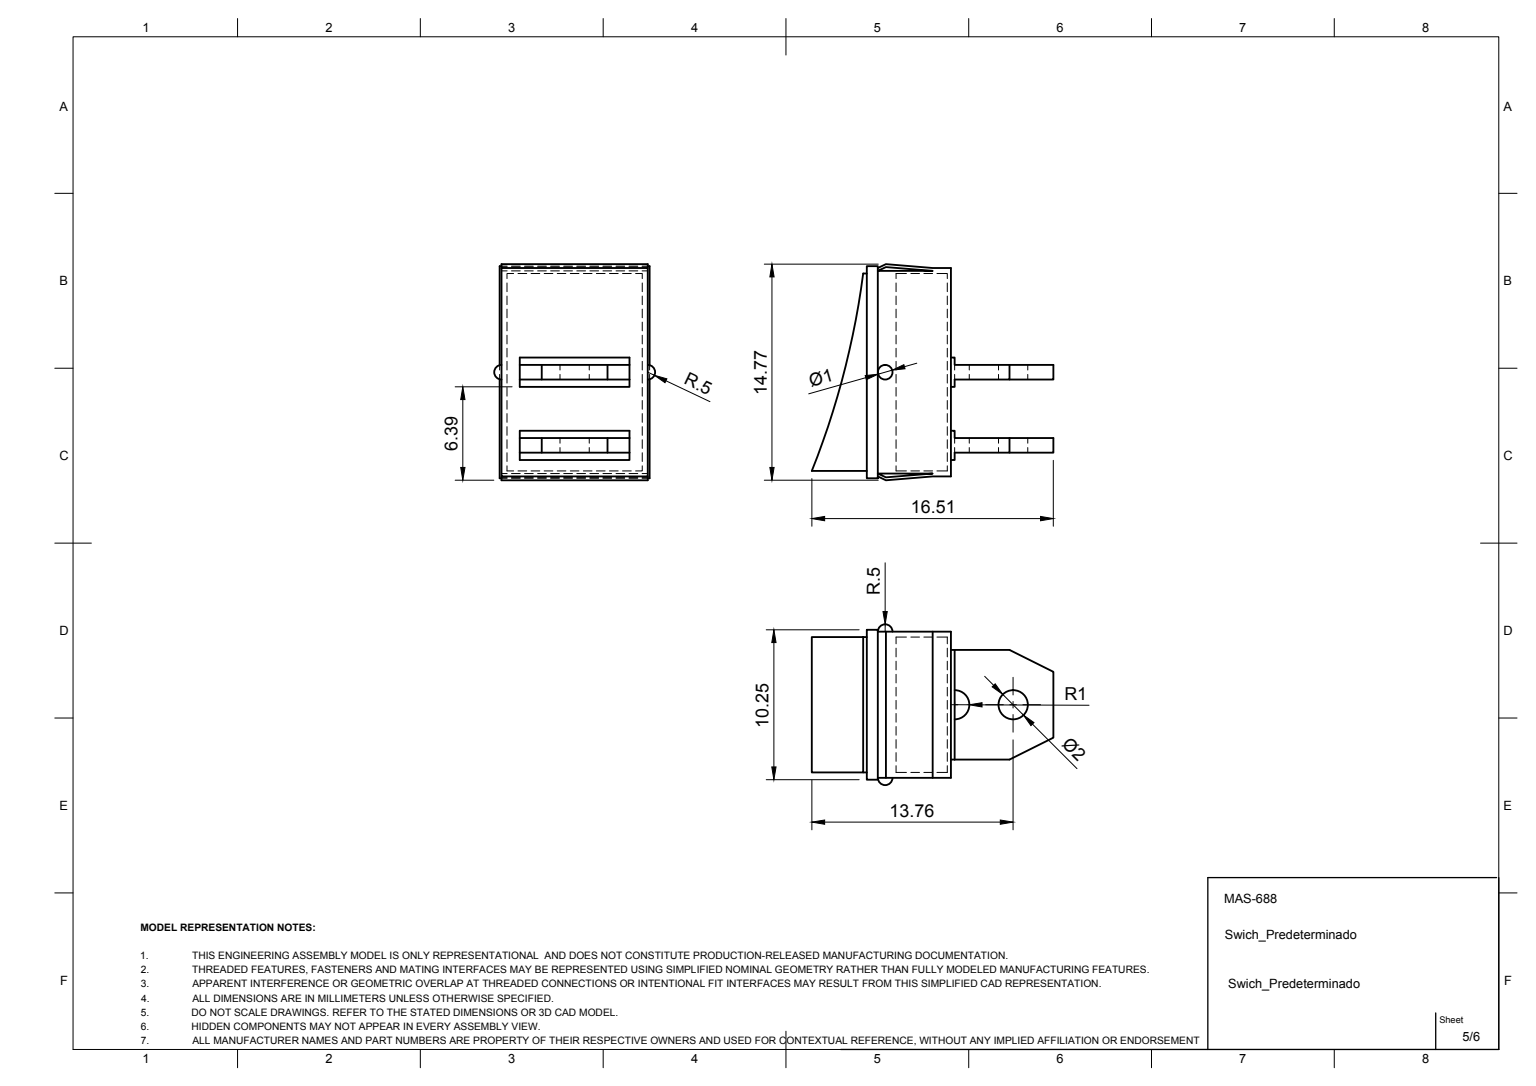
ISO-10303-21;
HEADER;
/* Generated by software containing ST-Developer
 * from STEP Tools, Inc. (www.steptools.com) 
 */

FILE_DESCRIPTION(
/* description */ ('STEP AP214'),
/* implementation_level */ '2;1');

FILE_NAME(
/* name */ 'Swich_Predeterminado.step',
/* time_stamp */ '2026-11-14T03:58:36-08:00',
/* author */ (''),
/* organization */ (''),
/* preprocessor_version */ 'ST-DEVELOPER v20.2',
/* originating_system */ 'Autodesk Translation Framework v15.17.0.0',
/* authorisation */ '');

FILE_SCHEMA (('AUTOMOTIVE_DESIGN { 1 0 10303 214 3 1 1 }'));
ENDSEC;

DATA;
#10=MECHANICAL_DESIGN_GEOMETRIC_PRESENTATION_REPRESENTATION('',(#43),#65304);
#27=SPHERICAL_SURFACE('',#41303,0.5);
#28=SPHERICAL_SURFACE('',#41305,0.5);
#29=ORIENTED_CLOSED_SHELL('',*,#39935,.F.);
#30=BREP_WITH_VOIDS('Body1',#39936,(#29));
#35=SHAPE_REPRESENTATION_RELATIONSHIP('SRR','None',#65326,#39);
#39=ADVANCED_BREP_SHAPE_REPRESENTATION('',(#30),#65302);
#43=STYLED_ITEM('',(#65355),#30);
#247=FACE_BOUND('',#5142,.T.);
#248=FACE_BOUND('',#5143,.T.);
#249=FACE_BOUND('',#5145,.T.);
#250=FACE_BOUND('',#5151,.T.);
#251=FACE_BOUND('',#5167,.T.);
#252=FACE_BOUND('',#5169,.T.);
#253=FACE_BOUND('',#5172,.T.);
#254=FACE_BOUND('',#5174,.T.);
#970=PLANE('',#41225);
#971=PLANE('',#41226);
#972=PLANE('',#41227);
#973=PLANE('',#41228);
#974=PLANE('',#41229);
#975=PLANE('',#41230);
#976=PLANE('',#41240);
#977=PLANE('',#41241);
#978=PLANE('',#41242);
#979=PLANE('',#41243);
#980=PLANE('',#41244);
#981=PLANE('',#41245);
#982=PLANE('',#41246);
#983=PLANE('',#41247);
#984=PLANE('',#41248);
#985=PLANE('',#41249);
#986=PLANE('',#41250);
#987=PLANE('',#41251);
#988=PLANE('',#41252);
#989=PLANE('',#41253);
#990=PLANE('',#41254);
#991=PLANE('',#41255);
#992=PLANE('',#41258);
#993=PLANE('',#41259);
#994=PLANE('',#41262);
#995=PLANE('',#41263);
#996=PLANE('',#41264);
#997=PLANE('',#41265);
#998=PLANE('',#41266);
#999=PLANE('',#41267);
#1000=PLANE('',#41268);
#1001=PLANE('',#41269);
#1002=PLANE('',#41270);
#1003=PLANE('',#41271);
#1004=PLANE('',#41272);
#1005=PLANE('',#41273);
#1006=PLANE('',#41275);
#1007=PLANE('',#41277);
#1008=PLANE('',#41278);
#1009=PLANE('',#41280);
#1010=PLANE('',#41282);
#1011=PLANE('',#41283);
#1012=PLANE('',#41284);
#1013=PLANE('',#41285);
#1014=PLANE('',#41286);
#1015=PLANE('',#41289);
#1016=PLANE('',#41290);
#1017=PLANE('',#41291);
#1018=PLANE('',#41292);
#1019=PLANE('',#41293);
#1020=PLANE('',#41294);
#1021=PLANE('',#41295);
#1022=PLANE('',#41296);
#1023=PLANE('',#41297);
#1024=PLANE('',#41298);
#1025=PLANE('',#41299);
#1026=PLANE('',#41300);
#1027=PLANE('',#41301);
#1028=PLANE('',#41302);
#3011=FACE_OUTER_BOUND('',#5124,.T.);
#3012=FACE_OUTER_BOUND('',#5125,.T.);
#3013=FACE_OUTER_BOUND('',#5126,.T.);
#3014=FACE_OUTER_BOUND('',#5127,.T.);
#3015=FACE_OUTER_BOUND('',#5128,.T.);
#3016=FACE_OUTER_BOUND('',#5129,.T.);
#3017=FACE_OUTER_BOUND('',#5130,.T.);
#3018=FACE_OUTER_BOUND('',#5131,.T.);
#3019=FACE_OUTER_BOUND('',#5132,.T.);
#3020=FACE_OUTER_BOUND('',#5133,.T.);
#3021=FACE_OUTER_BOUND('',#5134,.T.);
#3022=FACE_OUTER_BOUND('',#5135,.T.);
#3023=FACE_OUTER_BOUND('',#5136,.T.);
#3024=FACE_OUTER_BOUND('',#5137,.T.);
#3025=FACE_OUTER_BOUND('',#5138,.T.);
#3026=FACE_OUTER_BOUND('',#5139,.T.);
#3027=FACE_OUTER_BOUND('',#5140,.T.);
#3028=FACE_OUTER_BOUND('',#5141,.T.);
#3029=FACE_OUTER_BOUND('',#5144,.T.);
#3030=FACE_OUTER_BOUND('',#5146,.T.);
#3031=FACE_OUTER_BOUND('',#5147,.T.);
#3032=FACE_OUTER_BOUND('',#5148,.T.);
#3033=FACE_OUTER_BOUND('',#5149,.T.);
#3034=FACE_OUTER_BOUND('',#5150,.T.);
#3035=FACE_OUTER_BOUND('',#5152,.T.);
#3036=FACE_OUTER_BOUND('',#5153,.T.);
#3037=FACE_OUTER_BOUND('',#5154,.T.);
#3038=FACE_OUTER_BOUND('',#5155,.T.);
#3039=FACE_OUTER_BOUND('',#5156,.T.);
#3040=FACE_OUTER_BOUND('',#5157,.T.);
#3041=FACE_OUTER_BOUND('',#5158,.T.);
#3042=FACE_OUTER_BOUND('',#5159,.T.);
#3043=FACE_OUTER_BOUND('',#5160,.T.);
#3044=FACE_OUTER_BOUND('',#5161,.T.);
#3045=FACE_OUTER_BOUND('',#5162,.T.);
#3046=FACE_OUTER_BOUND('',#5163,.T.);
#3047=FACE_OUTER_BOUND('',#5164,.T.);
#3048=FACE_OUTER_BOUND('',#5165,.T.);
#3049=FACE_OUTER_BOUND('',#5166,.T.);
#3050=FACE_OUTER_BOUND('',#5168,.T.);
#3051=FACE_OUTER_BOUND('',#5170,.T.);
#3052=FACE_OUTER_BOUND('',#5171,.T.);
#3053=FACE_OUTER_BOUND('',#5173,.T.);
#3054=FACE_OUTER_BOUND('',#5175,.T.);
#3055=FACE_OUTER_BOUND('',#5176,.T.);
#3056=FACE_OUTER_BOUND('',#5177,.T.);
#3057=FACE_OUTER_BOUND('',#5178,.T.);
#3058=FACE_OUTER_BOUND('',#5179,.T.);
#3059=FACE_OUTER_BOUND('',#5180,.T.);
#3060=FACE_OUTER_BOUND('',#5181,.T.);
#3061=FACE_OUTER_BOUND('',#5182,.T.);
#3062=FACE_OUTER_BOUND('',#5183,.T.);
#3063=FACE_OUTER_BOUND('',#5184,.T.);
#3064=FACE_OUTER_BOUND('',#5185,.T.);
#3065=FACE_OUTER_BOUND('',#5186,.T.);
#3066=FACE_OUTER_BOUND('',#5187,.T.);
#3067=FACE_OUTER_BOUND('',#5188,.T.);
#3068=FACE_OUTER_BOUND('',#5189,.T.);
#3069=FACE_OUTER_BOUND('',#5190,.T.);
#3070=FACE_OUTER_BOUND('',#5191,.T.);
#3071=FACE_OUTER_BOUND('',#5192,.T.);
#3072=FACE_OUTER_BOUND('',#5193,.T.);
#3073=FACE_OUTER_BOUND('',#5194,.T.);
#3074=FACE_OUTER_BOUND('',#5195,.T.);
#3075=FACE_OUTER_BOUND('',#5196,.T.);
#3076=FACE_OUTER_BOUND('',#5197,.T.);
#5124=EDGE_LOOP('',(#30411,#30412,#30413,#30414));
#5125=EDGE_LOOP('',(#30415,#30416,#30417,#30418));
#5126=EDGE_LOOP('',(#30419,#30420,#30421,#30422));
#5127=EDGE_LOOP('',(#30423,#30424,#30425,#30426));
#5128=EDGE_LOOP('',(#30427,#30428,#30429,#30430));
#5129=EDGE_LOOP('',(#30431,#30432,#30433,#30434));
#5130=EDGE_LOOP('',(#30435,#30436,#30437,#30438));
#5131=EDGE_LOOP('',(#30439,#30440,#30441,#30442));
#5132=EDGE_LOOP('',(#30443,#30444,#30445,#30446));
#5133=EDGE_LOOP('',(#30447,#30448,#30449,#30450));
#5134=EDGE_LOOP('',(#30451,#30452,#30453,#30454));
#5135=EDGE_LOOP('',(#30455,#30456,#30457,#30458,#30459,#30460));
#5136=EDGE_LOOP('',(#30461,#30462,#30463,#30464,#30465,#30466));
#5137=EDGE_LOOP('',(#30467,#30468,#30469,#30470));
#5138=EDGE_LOOP('',(#30471,#30472,#30473,#30474));
#5139=EDGE_LOOP('',(#30475,#30476,#30477,#30478,#30479,#30480));
#5140=EDGE_LOOP('',(#30481,#30482,#30483,#30484,#30485,#30486));
#5141=EDGE_LOOP('',(#30487,#30488,#30489,#30490));
#5142=EDGE_LOOP('',(#30491,#30492,#30493,#30494,#30495,#30496,#30497,#30498));
#5143=EDGE_LOOP('',(#30499,#30500,#30501,#30502,#30503,#30504,#30505,#30506));
#5144=EDGE_LOOP('',(#30507,#30508,#30509,#30510));
#5145=EDGE_LOOP('',(#30511,#30512,#30513,#30514,#30515,#30516,#30517,#30518,
#30519,#30520));
#5146=EDGE_LOOP('',(#30521,#30522,#30523,#30524));
#5147=EDGE_LOOP('',(#30525,#30526,#30527,#30528));
#5148=EDGE_LOOP('',(#30529,#30530,#30531,#30532));
#5149=EDGE_LOOP('',(#30533,#30534,#30535,#30536));
#5150=EDGE_LOOP('',(#30537,#30538,#30539,#30540));
#5151=EDGE_LOOP('',(#30541,#30542,#30543,#30544));
#5152=EDGE_LOOP('',(#30545,#30546,#30547,#30548,#30549,#30550,#30551,#30552,
#30553,#30554,#30555,#30556,#30557,#30558,#30559,#30560,#30561,#30562,#30563));
#5153=EDGE_LOOP('',(#30564,#30565,#30566,#30567));
#5154=EDGE_LOOP('',(#30568,#30569,#30570,#30571,#30572,#30573,#30574,#30575,
#30576,#30577,#30578,#30579,#30580,#30581,#30582,#30583,#30584,#30585,#30586));
#5155=EDGE_LOOP('',(#30587,#30588,#30589,#30590));
#5156=EDGE_LOOP('',(#30591,#30592,#30593,#30594));
#5157=EDGE_LOOP('',(#30595,#30596,#30597,#30598));
#5158=EDGE_LOOP('',(#30599,#30600,#30601,#30602));
#5159=EDGE_LOOP('',(#30603,#30604,#30605,#30606,#30607,#30608,#30609,#30610,
#30611,#30612,#30613,#30614));
#5160=EDGE_LOOP('',(#30615,#30616,#30617,#30618));
#5161=EDGE_LOOP('',(#30619,#30620,#30621,#30622));
#5162=EDGE_LOOP('',(#30623,#30624,#30625,#30626));
#5163=EDGE_LOOP('',(#30627,#30628,#30629,#30630));
#5164=EDGE_LOOP('',(#30631,#30632,#30633,#30634,#30635,#30636,#30637,#30638,
#30639,#30640,#30641,#30642));
#5165=EDGE_LOOP('',(#30643,#30644,#30645,#30646));
#5166=EDGE_LOOP('',(#30647,#30648,#30649,#30650,#30651,#30652,#30653,#30654));
#5167=EDGE_LOOP('',(#30655));
#5168=EDGE_LOOP('',(#30656,#30657,#30658,#30659,#30660,#30661,#30662,#30663));
#5169=EDGE_LOOP('',(#30664));
#5170=EDGE_LOOP('',(#30665,#30666,#30667,#30668));
#5171=EDGE_LOOP('',(#30669,#30670,#30671,#30672,#30673,#30674,#30675,#30676));
#5172=EDGE_LOOP('',(#30677));
#5173=EDGE_LOOP('',(#30678,#30679,#30680,#30681,#30682,#30683,#30684,#30685));
#5174=EDGE_LOOP('',(#30686));
#5175=EDGE_LOOP('',(#30687,#30688,#30689,#30690));
#5176=EDGE_LOOP('',(#30691,#30692,#30693,#30694));
#5177=EDGE_LOOP('',(#30695,#30696,#30697,#30698));
#5178=EDGE_LOOP('',(#30699,#30700,#30701,#30702));
#5179=EDGE_LOOP('',(#30703,#30704,#30705,#30706));
#5180=EDGE_LOOP('',(#30707,#30708,#30709,#30710));
#5181=EDGE_LOOP('',(#30711,#30712,#30713,#30714));
#5182=EDGE_LOOP('',(#30715,#30716,#30717,#30718));
#5183=EDGE_LOOP('',(#30719,#30720,#30721,#30722));
#5184=EDGE_LOOP('',(#30723,#30724,#30725,#30726));
#5185=EDGE_LOOP('',(#30727,#30728,#30729,#30730));
#5186=EDGE_LOOP('',(#30731,#30732,#30733,#30734));
#5187=EDGE_LOOP('',(#30735,#30736,#30737,#30738));
#5188=EDGE_LOOP('',(#30739,#30740,#30741,#30742));
#5189=EDGE_LOOP('',(#30743,#30744,#30745,#30746));
#5190=EDGE_LOOP('',(#30747,#30748,#30749,#30750));
#5191=EDGE_LOOP('',(#30751,#30752,#30753,#30754));
#5192=EDGE_LOOP('',(#30755,#30756,#30757,#30758));
#5193=EDGE_LOOP('',(#30759,#30760,#30761,#30762));
#5194=EDGE_LOOP('',(#30763,#30764,#30765,#30766));
#5195=EDGE_LOOP('',(#30767,#30768,#30769,#30770));
#5196=EDGE_LOOP('',(#30771,#30772,#30773,#30774));
#5197=EDGE_LOOP('',(#30775,#30776,#30777,#30778));
#8011=LINE('',#57983,#12886);
#8012=LINE('',#57985,#12887);
#8013=LINE('',#57987,#12888);
#8014=LINE('',#57988,#12889);
#8015=LINE('',#57992,#12890);
#8016=LINE('',#57994,#12891);
#8017=LINE('',#57996,#12892);
#8018=LINE('',#57997,#12893);
#8019=LINE('',#57999,#12894);
#8020=LINE('',#58000,#12895);
#8021=LINE('',#58002,#12896);
#8022=LINE('',#58004,#12897);
#8023=LINE('',#58010,#12898);
#8024=LINE('',#58016,#12899);
#8025=LINE('',#58023,#12900);
#8026=LINE('',#58026,#12901);
#8027=LINE('',#58030,#12902);
#8028=LINE('',#58032,#12903);
#8029=LINE('',#58034,#12904);
#8030=LINE('',#58035,#12905);
#8031=LINE('',#58039,#12906);
#8032=LINE('',#58041,#12907);
#8033=LINE('',#58043,#12908);
#8034=LINE('',#58044,#12909);
#8035=LINE('',#58047,#12910);
#8036=LINE('',#58049,#12911);
#8037=LINE('',#58051,#12912);
#8038=LINE('',#58053,#12913);
#8039=LINE('',#58054,#12914);
#8040=LINE('',#58057,#12915);
#8041=LINE('',#58059,#12916);
#8042=LINE('',#58061,#12917);
#8043=LINE('',#58063,#12918);
#8044=LINE('',#58064,#12919);
#8045=LINE('',#58068,#12920);
#8046=LINE('',#58070,#12921);
#8047=LINE('',#58072,#12922);
#8048=LINE('',#58073,#12923);
#8049=LINE('',#58077,#12924);
#8050=LINE('',#58079,#12925);
#8051=LINE('',#58081,#12926);
#8052=LINE('',#58082,#12927);
#8053=LINE('',#58085,#12928);
#8054=LINE('',#58087,#12929);
#8055=LINE('',#58089,#12930);
#8056=LINE('',#58091,#12931);
#8057=LINE('',#58092,#12932);
#8058=LINE('',#58095,#12933);
#8059=LINE('',#58097,#12934);
#8060=LINE('',#58099,#12935);
#8061=LINE('',#58101,#12936);
#8062=LINE('',#58102,#12937);
#8063=LINE('',#58106,#12938);
#8064=LINE('',#58108,#12939);
#8065=LINE('',#58110,#12940);
#8066=LINE('',#58111,#12941);
#8067=LINE('',#58114,#12942);
#8068=LINE('',#58115,#12943);
#8069=LINE('',#58116,#12944);
#8070=LINE('',#58117,#12945);
#8071=LINE('',#58120,#12946);
#8072=LINE('',#58121,#12947);
#8073=LINE('',#58122,#12948);
#8074=LINE('',#58123,#12949);
#8075=LINE('',#58127,#12950);
#8076=LINE('',#58129,#12951);
#8077=LINE('',#58131,#12952);
#8078=LINE('',#58132,#12953);
#8079=LINE('',#58135,#12954);
#8080=LINE('',#58137,#12955);
#8081=LINE('',#58139,#12956);
#8082=LINE('',#58141,#12957);
#8083=LINE('',#58143,#12958);
#8084=LINE('',#58145,#12959);
#8085=LINE('',#58147,#12960);
#8086=LINE('',#58149,#12961);
#8087=LINE('',#58151,#12962);
#8088=LINE('',#58152,#12963);
#8089=LINE('',#58155,#12964);
#8090=LINE('',#58157,#12965);
#8091=LINE('',#58158,#12966);
#8092=LINE('',#58161,#12967);
#8093=LINE('',#58162,#12968);
#8094=LINE('',#58165,#12969);
#8095=LINE('',#58166,#12970);
#8096=LINE('',#58168,#12971);
#8097=LINE('',#58172,#12972);
#8098=LINE('',#58174,#12973);
#8099=LINE('',#58176,#12974);
#8100=LINE('',#58177,#12975);
#8101=LINE('',#58183,#12976);
#8102=LINE('',#58185,#12977);
#8103=LINE('',#58186,#12978);
#8104=LINE('',#58188,#12979);
#8105=LINE('',#58190,#12980);
#8106=LINE('',#58191,#12981);
#8107=LINE('',#58193,#12982);
#8108=LINE('',#58195,#12983);
#8109=LINE('',#58196,#12984);
#8110=LINE('',#58198,#12985);
#8111=LINE('',#58200,#12986);
#8112=LINE('',#58201,#12987);
#8113=LINE('',#58204,#12988);
#8114=LINE('',#58205,#12989);
#8115=LINE('',#58211,#12990);
#8116=LINE('',#58213,#12991);
#8117=LINE('',#58214,#12992);
#8118=LINE('',#58216,#12993);
#8119=LINE('',#58218,#12994);
#8120=LINE('',#58219,#12995);
#8121=LINE('',#58221,#12996);
#8122=LINE('',#58222,#12997);
#8123=LINE('',#58224,#12998);
#8124=LINE('',#58226,#12999);
#8125=LINE('',#58227,#13000);
#8126=LINE('',#58229,#13001);
#8127=LINE('',#58231,#13002);
#8128=LINE('',#58234,#13003);
#8129=LINE('',#58235,#13004);
#8130=LINE('',#58238,#13005);
#8131=LINE('',#58239,#13006);
#8132=LINE('',#58242,#13007);
#8133=LINE('',#58244,#13008);
#8134=LINE('',#58245,#13009);
#8135=LINE('',#58246,#13010);
#8136=LINE('',#58248,#13011);
#8137=LINE('',#58250,#13012);
#8138=LINE('',#58251,#13013);
#8139=LINE('',#58254,#13014);
#8140=LINE('',#58257,#13015);
#8141=LINE('',#58258,#13016);
#8142=LINE('',#58261,#13017);
#8143=LINE('',#58262,#13018);
#8144=LINE('',#58265,#13019);
#8145=LINE('',#58267,#13020);
#8146=LINE('',#58268,#13021);
#8147=LINE('',#58269,#13022);
#8148=LINE('',#58271,#13023);
#8149=LINE('',#58273,#13024);
#8150=LINE('',#58274,#13025);
#8151=LINE('',#58279,#13026);
#8152=LINE('',#58281,#13027);
#8153=LINE('',#58282,#13028);
#8154=LINE('',#58286,#13029);
#8155=LINE('',#58288,#13030);
#8156=LINE('',#58289,#13031);
#8157=LINE('',#58291,#13032);
#8158=LINE('',#58292,#13033);
#8159=LINE('',#58296,#13034);
#8160=LINE('',#58298,#13035);
#8161=LINE('',#58299,#13036);
#8162=LINE('',#58303,#13037);
#8163=LINE('',#58305,#13038);
#8164=LINE('',#58306,#13039);
#8165=LINE('',#58308,#13040);
#8166=LINE('',#58309,#13041);
#8167=LINE('',#58317,#13042);
#8168=LINE('',#58318,#13043);
#8169=LINE('',#58320,#13044);
#8170=LINE('',#58321,#13045);
#8171=LINE('',#58323,#13046);
#8172=LINE('',#58326,#13047);
#8173=LINE('',#58329,#13048);
#8174=LINE('',#58332,#13049);
#8175=LINE('',#58335,#13050);
#8176=LINE('',#58336,#13051);
#8177=LINE('',#58338,#13052);
#8178=LINE('',#58340,#13053);
#12886=VECTOR('',#46271,1000.);
#12887=VECTOR('',#46272,1000.);
#12888=VECTOR('',#46273,1000.);
#12889=VECTOR('',#46274,1000.);
#12890=VECTOR('',#46277,1000.);
#12891=VECTOR('',#46278,1000.);
#12892=VECTOR('',#46279,1000.);
#12893=VECTOR('',#46280,1000.);
#12894=VECTOR('',#46283,1000.);
#12895=VECTOR('',#46284,1000.);
#12896=VECTOR('',#46287,1000.);
#12897=VECTOR('',#46290,1000.);
#12898=VECTOR('',#46297,1.);
#12899=VECTOR('',#46304,1.);
#12900=VECTOR('',#46311,1000.);
#12901=VECTOR('',#46314,1000.);
#12902=VECTOR('',#46317,1000.);
#12903=VECTOR('',#46318,1000.);
#12904=VECTOR('',#46319,1000.);
#12905=VECTOR('',#46320,1000.);
#12906=VECTOR('',#46323,1000.);
#12907=VECTOR('',#46324,1000.);
#12908=VECTOR('',#46325,1000.);
#12909=VECTOR('',#46326,1000.);
#12910=VECTOR('',#46329,1000.);
#12911=VECTOR('',#46330,1000.);
#12912=VECTOR('',#46331,1000.);
#12913=VECTOR('',#46332,1000.);
#12914=VECTOR('',#46333,1000.);
#12915=VECTOR('',#46336,1000.);
#12916=VECTOR('',#46337,1000.);
#12917=VECTOR('',#46338,1000.);
#12918=VECTOR('',#46339,1000.);
#12919=VECTOR('',#46340,1000.);
#12920=VECTOR('',#46343,1000.);
#12921=VECTOR('',#46344,1000.);
#12922=VECTOR('',#46345,1000.);
#12923=VECTOR('',#46346,1000.);
#12924=VECTOR('',#46349,1000.);
#12925=VECTOR('',#46350,1000.);
#12926=VECTOR('',#46351,1000.);
#12927=VECTOR('',#46352,1000.);
#12928=VECTOR('',#46355,1000.);
#12929=VECTOR('',#46356,1000.);
#12930=VECTOR('',#46357,1000.);
#12931=VECTOR('',#46358,1000.);
#12932=VECTOR('',#46359,1000.);
#12933=VECTOR('',#46362,1000.);
#12934=VECTOR('',#46363,1000.);
#12935=VECTOR('',#46364,1000.);
#12936=VECTOR('',#46365,1000.);
#12937=VECTOR('',#46366,1000.);
#12938=VECTOR('',#46369,1000.);
#12939=VECTOR('',#46370,1000.);
#12940=VECTOR('',#46371,1000.);
#12941=VECTOR('',#46372,1000.);
#12942=VECTOR('',#46373,1000.);
#12943=VECTOR('',#46374,1000.);
#12944=VECTOR('',#46375,1000.);
#12945=VECTOR('',#46376,1000.);
#12946=VECTOR('',#46377,1000.);
#12947=VECTOR('',#46378,1000.);
#12948=VECTOR('',#46379,1000.);
#12949=VECTOR('',#46380,1000.);
#12950=VECTOR('',#46383,1000.);
#12951=VECTOR('',#46384,1000.);
#12952=VECTOR('',#46385,1000.);
#12953=VECTOR('',#46386,1000.);
#12954=VECTOR('',#46387,1000.);
#12955=VECTOR('',#46388,1000.);
#12956=VECTOR('',#46389,1000.);
#12957=VECTOR('',#46390,1000.);
#12958=VECTOR('',#46391,1000.);
#12959=VECTOR('',#46392,1000.);
#12960=VECTOR('',#46393,1000.);
#12961=VECTOR('',#46394,1000.);
#12962=VECTOR('',#46395,1000.);
#12963=VECTOR('',#46396,1000.);
#12964=VECTOR('',#46399,1000.);
#12965=VECTOR('',#46400,1000.);
#12966=VECTOR('',#46401,1000.);
#12967=VECTOR('',#46404,1000.);
#12968=VECTOR('',#46405,1000.);
#12969=VECTOR('',#46408,1000.);
#12970=VECTOR('',#46409,1000.);
#12971=VECTOR('',#46412,1000.);
#12972=VECTOR('',#46415,1000.);
#12973=VECTOR('',#46416,1000.);
#12974=VECTOR('',#46417,1000.);
#12975=VECTOR('',#46418,1000.);
#12976=VECTOR('',#46425,1000.);
#12977=VECTOR('',#46426,1000.);
#12978=VECTOR('',#46427,1000.);
#12979=VECTOR('',#46428,1000.);
#12980=VECTOR('',#46429,1000.);
#12981=VECTOR('',#46430,1000.);
#12982=VECTOR('',#46431,1000.);
#12983=VECTOR('',#46432,1000.);
#12984=VECTOR('',#46433,1000.);
#12985=VECTOR('',#46434,1000.);
#12986=VECTOR('',#46435,1000.);
#12987=VECTOR('',#46436,1000.);
#12988=VECTOR('',#46439,1000.);
#12989=VECTOR('',#46440,1000.);
#12990=VECTOR('',#46447,1000.);
#12991=VECTOR('',#46448,1000.);
#12992=VECTOR('',#46449,1000.);
#12993=VECTOR('',#46450,1000.);
#12994=VECTOR('',#46451,1000.);
#12995=VECTOR('',#46452,1000.);
#12996=VECTOR('',#46453,1000.);
#12997=VECTOR('',#46454,1000.);
#12998=VECTOR('',#46455,1000.);
#12999=VECTOR('',#46456,1000.);
#13000=VECTOR('',#46457,1000.);
#13001=VECTOR('',#46460,1000.);
#13002=VECTOR('',#46463,1000.);
#13003=VECTOR('',#46466,1000.);
#13004=VECTOR('',#46467,1000.);
#13005=VECTOR('',#46470,1000.);
#13006=VECTOR('',#46471,1000.);
#13007=VECTOR('',#46474,1000.);
#13008=VECTOR('',#46475,1000.);
#13009=VECTOR('',#46476,1000.);
#13010=VECTOR('',#46477,1000.);
#13011=VECTOR('',#46478,1000.);
#13012=VECTOR('',#46479,1000.);
#13013=VECTOR('',#46480,1000.);
#13014=VECTOR('',#46485,1000.);
#13015=VECTOR('',#46488,1000.);
#13016=VECTOR('',#46489,1000.);
#13017=VECTOR('',#46492,1000.);
#13018=VECTOR('',#46493,1000.);
#13019=VECTOR('',#46496,1000.);
#13020=VECTOR('',#46497,1000.);
#13021=VECTOR('',#46498,1000.);
#13022=VECTOR('',#46499,1000.);
#13023=VECTOR('',#46500,1000.);
#13024=VECTOR('',#46501,1000.);
#13025=VECTOR('',#46502,1000.);
#13026=VECTOR('',#46509,1000.);
#13027=VECTOR('',#46510,1000.);
#13028=VECTOR('',#46511,1000.);
#13029=VECTOR('',#46516,1000.);
#13030=VECTOR('',#46517,1000.);
#13031=VECTOR('',#46518,1000.);
#13032=VECTOR('',#46521,1000.);
#13033=VECTOR('',#46522,1000.);
#13034=VECTOR('',#46527,1000.);
#13035=VECTOR('',#46528,1000.);
#13036=VECTOR('',#46529,1000.);
#13037=VECTOR('',#46534,1000.);
#13038=VECTOR('',#46535,1000.);
#13039=VECTOR('',#46536,1000.);
#13040=VECTOR('',#46539,1000.);
#13041=VECTOR('',#46540,1000.);
#13042=VECTOR('',#46555,1000.);
#13043=VECTOR('',#46556,1000.);
#13044=VECTOR('',#46559,1000.);
#13045=VECTOR('',#46560,1000.);
#13046=VECTOR('',#46563,1000.);
#13047=VECTOR('',#46568,1000.);
#13048=VECTOR('',#46573,1000.);
#13049=VECTOR('',#46578,1000.);
#13050=VECTOR('',#46583,1000.);
#13051=VECTOR('',#46584,1000.);
#13052=VECTOR('',#46587,1000.);
#13053=VECTOR('',#46590,1000.);
#17094=CIRCLE('',#41232,1.);
#17095=CIRCLE('',#41233,1.);
#17096=CIRCLE('',#41235,1.);
#17097=CIRCLE('',#41236,1.);
#17098=CIRCLE('',#41238,56.);
#17099=CIRCLE('',#41239,56.);
#17100=CIRCLE('',#41256,0.5);
#17101=CIRCLE('',#41257,0.5);
#17102=CIRCLE('',#41260,0.5);
#17103=CIRCLE('',#41261,0.5);
#17104=CIRCLE('',#41274,1.);
#17105=CIRCLE('',#41276,1.);
#17106=CIRCLE('',#41279,1.);
#17107=CIRCLE('',#41281,1.);
#17108=CIRCLE('',#41304,0.5);
#17109=CIRCLE('',#41306,0.5);
#18436=VERTEX_POINT('',#57981);
#18437=VERTEX_POINT('',#57982);
#18438=VERTEX_POINT('',#57984);
#18439=VERTEX_POINT('',#57986);
#18440=VERTEX_POINT('',#57990);
#18441=VERTEX_POINT('',#57991);
#18442=VERTEX_POINT('',#57993);
#18443=VERTEX_POINT('',#57995);
#18444=VERTEX_POINT('',#58007);
#18445=VERTEX_POINT('',#58009);
#18446=VERTEX_POINT('',#58013);
#18447=VERTEX_POINT('',#58015);
#18448=VERTEX_POINT('',#58019);
#18449=VERTEX_POINT('',#58020);
#18450=VERTEX_POINT('',#58022);
#18451=VERTEX_POINT('',#58024);
#18452=VERTEX_POINT('',#58028);
#18453=VERTEX_POINT('',#58029);
#18454=VERTEX_POINT('',#58031);
#18455=VERTEX_POINT('',#58033);
#18456=VERTEX_POINT('',#58037);
#18457=VERTEX_POINT('',#58038);
#18458=VERTEX_POINT('',#58040);
#18459=VERTEX_POINT('',#58042);
#18460=VERTEX_POINT('',#58046);
#18461=VERTEX_POINT('',#58048);
#18462=VERTEX_POINT('',#58050);
#18463=VERTEX_POINT('',#58052);
#18464=VERTEX_POINT('',#58056);
#18465=VERTEX_POINT('',#58058);
#18466=VERTEX_POINT('',#58060);
#18467=VERTEX_POINT('',#58062);
#18468=VERTEX_POINT('',#58066);
#18469=VERTEX_POINT('',#58067);
#18470=VERTEX_POINT('',#58069);
#18471=VERTEX_POINT('',#58071);
#18472=VERTEX_POINT('',#58075);
#18473=VERTEX_POINT('',#58076);
#18474=VERTEX_POINT('',#58078);
#18475=VERTEX_POINT('',#58080);
#18476=VERTEX_POINT('',#58084);
#18477=VERTEX_POINT('',#58086);
#18478=VERTEX_POINT('',#58088);
#18479=VERTEX_POINT('',#58090);
#18480=VERTEX_POINT('',#58094);
#18481=VERTEX_POINT('',#58096);
#18482=VERTEX_POINT('',#58098);
#18483=VERTEX_POINT('',#58100);
#18484=VERTEX_POINT('',#58104);
#18485=VERTEX_POINT('',#58105);
#18486=VERTEX_POINT('',#58107);
#18487=VERTEX_POINT('',#58109);
#18488=VERTEX_POINT('',#58112);
#18489=VERTEX_POINT('',#58113);
#18490=VERTEX_POINT('',#58118);
#18491=VERTEX_POINT('',#58119);
#18492=VERTEX_POINT('',#58125);
#18493=VERTEX_POINT('',#58126);
#18494=VERTEX_POINT('',#58128);
#18495=VERTEX_POINT('',#58130);
#18496=VERTEX_POINT('',#58133);
#18497=VERTEX_POINT('',#58134);
#18498=VERTEX_POINT('',#58136);
#18499=VERTEX_POINT('',#58138);
#18500=VERTEX_POINT('',#58140);
#18501=VERTEX_POINT('',#58142);
#18502=VERTEX_POINT('',#58144);
#18503=VERTEX_POINT('',#58146);
#18504=VERTEX_POINT('',#58148);
#18505=VERTEX_POINT('',#58150);
#18506=VERTEX_POINT('',#58154);
#18507=VERTEX_POINT('',#58156);
#18508=VERTEX_POINT('',#58160);
#18509=VERTEX_POINT('',#58164);
#18510=VERTEX_POINT('',#58170);
#18511=VERTEX_POINT('',#58171);
#18512=VERTEX_POINT('',#58173);
#18513=VERTEX_POINT('',#58175);
#18514=VERTEX_POINT('',#58179);
#18515=VERTEX_POINT('',#58182);
#18516=VERTEX_POINT('',#58184);
#18517=VERTEX_POINT('',#58187);
#18518=VERTEX_POINT('',#58189);
#18519=VERTEX_POINT('',#58192);
#18520=VERTEX_POINT('',#58194);
#18521=VERTEX_POINT('',#58197);
#18522=VERTEX_POINT('',#58199);
#18523=VERTEX_POINT('',#58203);
#18524=VERTEX_POINT('',#58207);
#18525=VERTEX_POINT('',#58210);
#18526=VERTEX_POINT('',#58212);
#18527=VERTEX_POINT('',#58215);
#18528=VERTEX_POINT('',#58217);
#18529=VERTEX_POINT('',#58220);
#18530=VERTEX_POINT('',#58223);
#18531=VERTEX_POINT('',#58225);
#18532=VERTEX_POINT('',#58233);
#18533=VERTEX_POINT('',#58237);
#18534=VERTEX_POINT('',#58241);
#18535=VERTEX_POINT('',#58243);
#18536=VERTEX_POINT('',#58247);
#18537=VERTEX_POINT('',#58249);
#18538=VERTEX_POINT('',#58256);
#18539=VERTEX_POINT('',#58260);
#18540=VERTEX_POINT('',#58264);
#18541=VERTEX_POINT('',#58266);
#18542=VERTEX_POINT('',#58270);
#18543=VERTEX_POINT('',#58272);
#18544=VERTEX_POINT('',#58278);
#18545=VERTEX_POINT('',#58280);
#18546=VERTEX_POINT('',#58285);
#18547=VERTEX_POINT('',#58287);
#18548=VERTEX_POINT('',#58295);
#18549=VERTEX_POINT('',#58297);
#18550=VERTEX_POINT('',#58302);
#18551=VERTEX_POINT('',#58304);
#18552=VERTEX_POINT('',#58343);
#18553=VERTEX_POINT('',#58346);
#22823=EDGE_CURVE('',#18436,#18437,#8011,.T.);
#22824=EDGE_CURVE('',#18438,#18436,#8012,.T.);
#22825=EDGE_CURVE('',#18439,#18438,#8013,.T.);
#22826=EDGE_CURVE('',#18437,#18439,#8014,.T.);
#22827=EDGE_CURVE('',#18440,#18441,#8015,.T.);
#22828=EDGE_CURVE('',#18441,#18442,#8016,.T.);
#22829=EDGE_CURVE('',#18442,#18443,#8017,.T.);
#22830=EDGE_CURVE('',#18443,#18440,#8018,.T.);
#22831=EDGE_CURVE('',#18441,#18439,#8019,.T.);
#22832=EDGE_CURVE('',#18440,#18437,#8020,.T.);
#22833=EDGE_CURVE('',#18443,#18436,#8021,.T.);
#22834=EDGE_CURVE('',#18442,#18438,#8022,.T.);
#22835=EDGE_CURVE('',#18444,#18444,#17094,.T.);
#22836=EDGE_CURVE('',#18444,#18445,#8023,.T.);
#22837=EDGE_CURVE('',#18445,#18445,#17095,.T.);
#22838=EDGE_CURVE('',#18446,#18446,#17096,.T.);
#22839=EDGE_CURVE('',#18446,#18447,#8024,.T.);
#22840=EDGE_CURVE('',#18447,#18447,#17097,.T.);
#22841=EDGE_CURVE('',#18448,#18449,#17098,.T.);
#22842=EDGE_CURVE('',#18448,#18450,#8025,.T.);
#22843=EDGE_CURVE('',#18450,#18451,#17099,.T.);
#22844=EDGE_CURVE('',#18451,#18449,#8026,.T.);
#22845=EDGE_CURVE('',#18452,#18453,#8027,.T.);
#22846=EDGE_CURVE('',#18454,#18452,#8028,.T.);
#22847=EDGE_CURVE('',#18454,#18455,#8029,.T.);
#22848=EDGE_CURVE('',#18455,#18453,#8030,.T.);
#22849=EDGE_CURVE('',#18456,#18457,#8031,.T.);
#22850=EDGE_CURVE('',#18457,#18458,#8032,.T.);
#22851=EDGE_CURVE('',#18459,#18458,#8033,.T.);
#22852=EDGE_CURVE('',#18456,#18459,#8034,.T.);
#22853=EDGE_CURVE('',#18460,#18452,#8035,.T.);
#22854=EDGE_CURVE('',#18453,#18461,#8036,.T.);
#22855=EDGE_CURVE('',#18462,#18461,#8037,.T.);
#22856=EDGE_CURVE('',#18463,#18462,#8038,.T.);
#22857=EDGE_CURVE('',#18460,#18463,#8039,.T.);
#22858=EDGE_CURVE('',#18464,#18457,#8040,.T.);
#22859=EDGE_CURVE('',#18464,#18465,#8041,.T.);
#22860=EDGE_CURVE('',#18465,#18466,#8042,.T.);
#22861=EDGE_CURVE('',#18466,#18467,#8043,.T.);
#22862=EDGE_CURVE('',#18458,#18467,#8044,.T.);
#22863=EDGE_CURVE('',#18468,#18469,#8045,.T.);
#22864=EDGE_CURVE('',#18469,#18470,#8046,.T.);
#22865=EDGE_CURVE('',#18471,#18470,#8047,.T.);
#22866=EDGE_CURVE('',#18468,#18471,#8048,.T.);
#22867=EDGE_CURVE('',#18472,#18473,#8049,.T.);
#22868=EDGE_CURVE('',#18474,#18472,#8050,.T.);
#22869=EDGE_CURVE('',#18474,#18475,#8051,.T.);
#22870=EDGE_CURVE('',#18475,#18473,#8052,.T.);
#22871=EDGE_CURVE('',#18476,#18469,#8053,.T.);
#22872=EDGE_CURVE('',#18476,#18477,#8054,.T.);
#22873=EDGE_CURVE('',#18477,#18478,#8055,.T.);
#22874=EDGE_CURVE('',#18478,#18479,#8056,.T.);
#22875=EDGE_CURVE('',#18470,#18479,#8057,.T.);
#22876=EDGE_CURVE('',#18480,#18472,#8058,.T.);
#22877=EDGE_CURVE('',#18473,#18481,#8059,.T.);
#22878=EDGE_CURVE('',#18482,#18481,#8060,.T.);
#22879=EDGE_CURVE('',#18483,#18482,#8061,.T.);
#22880=EDGE_CURVE('',#18480,#18483,#8062,.T.);
#22881=EDGE_CURVE('',#18484,#18485,#8063,.T.);
#22882=EDGE_CURVE('',#18485,#18486,#8064,.T.);
#22883=EDGE_CURVE('',#18486,#18487,#8065,.T.);
#22884=EDGE_CURVE('',#18487,#18484,#8066,.T.);
#22885=EDGE_CURVE('',#18488,#18489,#8067,.T.);
#22886=EDGE_CURVE('',#18461,#18488,#8068,.T.);
#22887=EDGE_CURVE('',#18455,#18459,#8069,.T.);
#22888=EDGE_CURVE('',#18467,#18489,#8070,.T.);
#22889=EDGE_CURVE('',#18490,#18491,#8071,.T.);
#22890=EDGE_CURVE('',#18481,#18490,#8072,.T.);
#22891=EDGE_CURVE('',#18475,#18471,#8073,.T.);
#22892=EDGE_CURVE('',#18479,#18491,#8074,.T.);
#22893=EDGE_CURVE('',#18492,#18493,#8075,.T.);
#22894=EDGE_CURVE('',#18494,#18493,#8076,.T.);
#22895=EDGE_CURVE('',#18495,#18494,#8077,.T.);
#22896=EDGE_CURVE('',#18495,#18492,#8078,.T.);
#22897=EDGE_CURVE('',#18496,#18497,#8079,.T.);
#22898=EDGE_CURVE('',#18498,#18496,#8080,.T.);
#22899=EDGE_CURVE('',#18499,#18498,#8081,.T.);
#22900=EDGE_CURVE('',#18500,#18499,#8082,.T.);
#22901=EDGE_CURVE('',#18500,#18501,#8083,.T.);
#22902=EDGE_CURVE('',#18501,#18502,#8084,.T.);
#22903=EDGE_CURVE('',#18503,#18502,#8085,.T.);
#22904=EDGE_CURVE('',#18504,#18503,#8086,.T.);
#22905=EDGE_CURVE('',#18505,#18504,#8087,.T.);
#22906=EDGE_CURVE('',#18505,#18497,#8088,.T.);
#22907=EDGE_CURVE('',#18506,#18494,#8089,.T.);
#22908=EDGE_CURVE('',#18507,#18506,#8090,.T.);
#22909=EDGE_CURVE('',#18507,#18495,#8091,.T.);
#22910=EDGE_CURVE('',#18508,#18493,#8092,.T.);
#22911=EDGE_CURVE('',#18506,#18508,#8093,.T.);
#22912=EDGE_CURVE('',#18509,#18492,#8094,.T.);
#22913=EDGE_CURVE('',#18509,#18508,#8095,.T.);
#22914=EDGE_CURVE('',#18507,#18509,#8096,.T.);
#22915=EDGE_CURVE('',#18510,#18511,#8097,.T.);
#22916=EDGE_CURVE('',#18512,#18510,#8098,.T.);
#22917=EDGE_CURVE('',#18513,#18512,#8099,.T.);
#22918=EDGE_CURVE('',#18511,#18513,#8100,.T.);
#22919=EDGE_CURVE('',#18514,#18504,#17100,.T.);
#22920=EDGE_CURVE('',#18504,#18514,#17101,.T.);
#22921=EDGE_CURVE('',#18503,#18515,#8101,.T.);
#22922=EDGE_CURVE('',#18515,#18516,#8102,.T.);
#22923=EDGE_CURVE('',#18516,#18503,#8103,.T.);
#22924=EDGE_CURVE('',#18502,#18517,#8104,.T.);
#22925=EDGE_CURVE('',#18517,#18518,#8105,.T.);
#22926=EDGE_CURVE('',#18485,#18518,#8106,.T.);
#22927=EDGE_CURVE('',#18484,#18519,#8107,.T.);
#22928=EDGE_CURVE('',#18520,#18519,#8108,.T.);
#22929=EDGE_CURVE('',#18497,#18520,#8109,.T.);
#22930=EDGE_CURVE('',#18521,#18505,#8110,.T.);
#22931=EDGE_CURVE('',#18522,#18521,#8111,.T.);
#22932=EDGE_CURVE('',#18522,#18505,#8112,.T.);
#22933=EDGE_CURVE('',#18523,#18518,#8113,.T.);
#22934=EDGE_CURVE('',#18486,#18523,#8114,.T.);
#22935=EDGE_CURVE('',#18524,#18499,#17102,.T.);
#22936=EDGE_CURVE('',#18499,#18524,#17103,.T.);
#22937=EDGE_CURVE('',#18498,#18525,#8115,.T.);
#22938=EDGE_CURVE('',#18525,#18526,#8116,.T.);
#22939=EDGE_CURVE('',#18526,#18498,#8117,.T.);
#22940=EDGE_CURVE('',#18496,#18527,#8118,.T.);
#22941=EDGE_CURVE('',#18527,#18528,#8119,.T.);
#22942=EDGE_CURVE('',#18487,#18528,#8120,.T.);
#22943=EDGE_CURVE('',#18529,#18523,#8121,.T.);
#22944=EDGE_CURVE('',#18501,#18529,#8122,.T.);
#22945=EDGE_CURVE('',#18530,#18500,#8123,.T.);
#22946=EDGE_CURVE('',#18531,#18530,#8124,.T.);
#22947=EDGE_CURVE('',#18531,#18500,#8125,.T.);
#22948=EDGE_CURVE('',#18528,#18519,#8126,.T.);
#22949=EDGE_CURVE('',#18454,#18456,#8127,.T.);
#22950=EDGE_CURVE('',#18462,#18532,#8128,.T.);
#22951=EDGE_CURVE('',#18532,#18488,#8129,.T.);
#22952=EDGE_CURVE('',#18466,#18533,#8130,.T.);
#22953=EDGE_CURVE('',#18533,#18489,#8131,.T.);
#22954=EDGE_CURVE('',#18452,#18534,#8132,.T.);
#22955=EDGE_CURVE('',#18535,#18534,#8133,.T.);
#22956=EDGE_CURVE('',#18462,#18535,#8134,.T.);
#22957=EDGE_CURVE('',#18532,#18533,#8135,.T.);
#22958=EDGE_CURVE('',#18536,#18466,#8136,.T.);
#22959=EDGE_CURVE('',#18536,#18537,#8137,.T.);
#22960=EDGE_CURVE('',#18537,#18457,#8138,.T.);
#22961=EDGE_CURVE('',#18474,#18468,#8139,.T.);
#22962=EDGE_CURVE('',#18482,#18538,#8140,.T.);
#22963=EDGE_CURVE('',#18538,#18490,#8141,.T.);
#22964=EDGE_CURVE('',#18478,#18539,#8142,.T.);
#22965=EDGE_CURVE('',#18539,#18491,#8143,.T.);
#22966=EDGE_CURVE('',#18472,#18540,#8144,.T.);
#22967=EDGE_CURVE('',#18541,#18540,#8145,.T.);
#22968=EDGE_CURVE('',#18482,#18541,#8146,.T.);
#22969=EDGE_CURVE('',#18538,#18539,#8147,.T.);
#22970=EDGE_CURVE('',#18542,#18478,#8148,.T.);
#22971=EDGE_CURVE('',#18542,#18543,#8149,.T.);
#22972=EDGE_CURVE('',#18543,#18469,#8150,.T.);
#22973=EDGE_CURVE('',#18534,#18537,#17104,.T.);
#22974=EDGE_CURVE('',#18544,#18460,#8151,.T.);
#22975=EDGE_CURVE('',#18544,#18545,#8152,.T.);
#22976=EDGE_CURVE('',#18464,#18545,#8153,.T.);
#22977=EDGE_CURVE('',#18535,#18536,#17105,.T.);
#22978=EDGE_CURVE('',#18465,#18546,#8154,.T.);
#22979=EDGE_CURVE('',#18547,#18546,#8155,.T.);
#22980=EDGE_CURVE('',#18547,#18463,#8156,.T.);
#22981=EDGE_CURVE('',#18545,#18546,#8157,.T.);
#22982=EDGE_CURVE('',#18544,#18547,#8158,.T.);
#22983=EDGE_CURVE('',#18540,#18543,#17106,.T.);
#22984=EDGE_CURVE('',#18548,#18480,#8159,.T.);
#22985=EDGE_CURVE('',#18548,#18549,#8160,.T.);
#22986=EDGE_CURVE('',#18476,#18549,#8161,.T.);
#22987=EDGE_CURVE('',#18541,#18542,#17107,.T.);
#22988=EDGE_CURVE('',#18550,#18477,#8162,.T.);
#22989=EDGE_CURVE('',#18551,#18550,#8163,.T.);
#22990=EDGE_CURVE('',#18483,#18551,#8164,.T.);
#22991=EDGE_CURVE('',#18549,#18550,#8165,.T.);
#22992=EDGE_CURVE('',#18551,#18548,#8166,.T.);
#22993=EDGE_CURVE('',#18525,#18522,#8167,.T.);
#22994=EDGE_CURVE('',#18498,#18505,#8168,.T.);
#22995=EDGE_CURVE('',#18500,#18503,#8169,.T.);
#22996=EDGE_CURVE('',#18531,#18515,#8170,.T.);
#22997=EDGE_CURVE('',#18530,#18516,#8171,.T.);
#22998=EDGE_CURVE('',#18529,#18517,#8172,.T.);
#22999=EDGE_CURVE('',#18527,#18520,#8173,.T.);
#23000=EDGE_CURVE('',#18526,#18521,#8174,.T.);
#23001=EDGE_CURVE('',#18450,#18512,#8175,.T.);
#23002=EDGE_CURVE('',#18448,#18513,#8176,.T.);
#23003=EDGE_CURVE('',#18451,#18510,#8177,.T.);
#23004=EDGE_CURVE('',#18449,#18511,#8178,.T.);
#23005=EDGE_CURVE('',#18514,#18552,#17108,.T.);
#23006=EDGE_CURVE('',#18524,#18553,#17109,.T.);
#30411=ORIENTED_EDGE('',*,*,#22823,.F.);
#30412=ORIENTED_EDGE('',*,*,#22824,.F.);
#30413=ORIENTED_EDGE('',*,*,#22825,.F.);
#30414=ORIENTED_EDGE('',*,*,#22826,.F.);
#30415=ORIENTED_EDGE('',*,*,#22827,.T.);
#30416=ORIENTED_EDGE('',*,*,#22828,.T.);
#30417=ORIENTED_EDGE('',*,*,#22829,.T.);
#30418=ORIENTED_EDGE('',*,*,#22830,.T.);
#30419=ORIENTED_EDGE('',*,*,#22826,.T.);
#30420=ORIENTED_EDGE('',*,*,#22831,.F.);
#30421=ORIENTED_EDGE('',*,*,#22827,.F.);
#30422=ORIENTED_EDGE('',*,*,#22832,.T.);
#30423=ORIENTED_EDGE('',*,*,#22823,.T.);
#30424=ORIENTED_EDGE('',*,*,#22832,.F.);
#30425=ORIENTED_EDGE('',*,*,#22830,.F.);
#30426=ORIENTED_EDGE('',*,*,#22833,.T.);
#30427=ORIENTED_EDGE('',*,*,#22824,.T.);
#30428=ORIENTED_EDGE('',*,*,#22833,.F.);
#30429=ORIENTED_EDGE('',*,*,#22829,.F.);
#30430=ORIENTED_EDGE('',*,*,#22834,.T.);
#30431=ORIENTED_EDGE('',*,*,#22825,.T.);
#30432=ORIENTED_EDGE('',*,*,#22834,.F.);
#30433=ORIENTED_EDGE('',*,*,#22828,.F.);
#30434=ORIENTED_EDGE('',*,*,#22831,.T.);
#30435=ORIENTED_EDGE('',*,*,#22835,.F.);
#30436=ORIENTED_EDGE('',*,*,#22836,.T.);
#30437=ORIENTED_EDGE('',*,*,#22837,.T.);
#30438=ORIENTED_EDGE('',*,*,#22836,.F.);
#30439=ORIENTED_EDGE('',*,*,#22838,.F.);
#30440=ORIENTED_EDGE('',*,*,#22839,.T.);
#30441=ORIENTED_EDGE('',*,*,#22840,.T.);
#30442=ORIENTED_EDGE('',*,*,#22839,.F.);
#30443=ORIENTED_EDGE('',*,*,#22841,.F.);
#30444=ORIENTED_EDGE('',*,*,#22842,.T.);
#30445=ORIENTED_EDGE('',*,*,#22843,.T.);
#30446=ORIENTED_EDGE('',*,*,#22844,.T.);
#30447=ORIENTED_EDGE('',*,*,#22845,.F.);
#30448=ORIENTED_EDGE('',*,*,#22846,.F.);
#30449=ORIENTED_EDGE('',*,*,#22847,.T.);
#30450=ORIENTED_EDGE('',*,*,#22848,.T.);
#30451=ORIENTED_EDGE('',*,*,#22849,.T.);
#30452=ORIENTED_EDGE('',*,*,#22850,.T.);
#30453=ORIENTED_EDGE('',*,*,#22851,.F.);
#30454=ORIENTED_EDGE('',*,*,#22852,.F.);
#30455=ORIENTED_EDGE('',*,*,#22853,.T.);
#30456=ORIENTED_EDGE('',*,*,#22845,.T.);
#30457=ORIENTED_EDGE('',*,*,#22854,.T.);
#30458=ORIENTED_EDGE('',*,*,#22855,.F.);
#30459=ORIENTED_EDGE('',*,*,#22856,.F.);
#30460=ORIENTED_EDGE('',*,*,#22857,.F.);
#30461=ORIENTED_EDGE('',*,*,#22850,.F.);
#30462=ORIENTED_EDGE('',*,*,#22858,.F.);
#30463=ORIENTED_EDGE('',*,*,#22859,.T.);
#30464=ORIENTED_EDGE('',*,*,#22860,.T.);
#30465=ORIENTED_EDGE('',*,*,#22861,.T.);
#30466=ORIENTED_EDGE('',*,*,#22862,.F.);
#30467=ORIENTED_EDGE('',*,*,#22863,.T.);
#30468=ORIENTED_EDGE('',*,*,#22864,.T.);
#30469=ORIENTED_EDGE('',*,*,#22865,.F.);
#30470=ORIENTED_EDGE('',*,*,#22866,.F.);
#30471=ORIENTED_EDGE('',*,*,#22867,.F.);
#30472=ORIENTED_EDGE('',*,*,#22868,.F.);
#30473=ORIENTED_EDGE('',*,*,#22869,.T.);
#30474=ORIENTED_EDGE('',*,*,#22870,.T.);
#30475=ORIENTED_EDGE('',*,*,#22864,.F.);
#30476=ORIENTED_EDGE('',*,*,#22871,.F.);
#30477=ORIENTED_EDGE('',*,*,#22872,.T.);
#30478=ORIENTED_EDGE('',*,*,#22873,.T.);
#30479=ORIENTED_EDGE('',*,*,#22874,.T.);
#30480=ORIENTED_EDGE('',*,*,#22875,.F.);
#30481=ORIENTED_EDGE('',*,*,#22876,.T.);
#30482=ORIENTED_EDGE('',*,*,#22867,.T.);
#30483=ORIENTED_EDGE('',*,*,#22877,.T.);
#30484=ORIENTED_EDGE('',*,*,#22878,.F.);
#30485=ORIENTED_EDGE('',*,*,#22879,.F.);
#30486=ORIENTED_EDGE('',*,*,#22880,.F.);
#30487=ORIENTED_EDGE('',*,*,#22881,.T.);
#30488=ORIENTED_EDGE('',*,*,#22882,.T.);
#30489=ORIENTED_EDGE('',*,*,#22883,.T.);
#30490=ORIENTED_EDGE('',*,*,#22884,.T.);
#30491=ORIENTED_EDGE('',*,*,#22885,.F.);
#30492=ORIENTED_EDGE('',*,*,#22886,.F.);
#30493=ORIENTED_EDGE('',*,*,#22854,.F.);
#30494=ORIENTED_EDGE('',*,*,#22848,.F.);
#30495=ORIENTED_EDGE('',*,*,#22887,.T.);
#30496=ORIENTED_EDGE('',*,*,#22851,.T.);
#30497=ORIENTED_EDGE('',*,*,#22862,.T.);
#30498=ORIENTED_EDGE('',*,*,#22888,.T.);
#30499=ORIENTED_EDGE('',*,*,#22889,.F.);
#30500=ORIENTED_EDGE('',*,*,#22890,.F.);
#30501=ORIENTED_EDGE('',*,*,#22877,.F.);
#30502=ORIENTED_EDGE('',*,*,#22870,.F.);
#30503=ORIENTED_EDGE('',*,*,#22891,.T.);
#30504=ORIENTED_EDGE('',*,*,#22865,.T.);
#30505=ORIENTED_EDGE('',*,*,#22875,.T.);
#30506=ORIENTED_EDGE('',*,*,#22892,.T.);
#30507=ORIENTED_EDGE('',*,*,#22893,.T.);
#30508=ORIENTED_EDGE('',*,*,#22894,.F.);
#30509=ORIENTED_EDGE('',*,*,#22895,.F.);
#30510=ORIENTED_EDGE('',*,*,#22896,.T.);
#30511=ORIENTED_EDGE('',*,*,#22897,.F.);
#30512=ORIENTED_EDGE('',*,*,#22898,.F.);
#30513=ORIENTED_EDGE('',*,*,#22899,.F.);
#30514=ORIENTED_EDGE('',*,*,#22900,.F.);
#30515=ORIENTED_EDGE('',*,*,#22901,.T.);
#30516=ORIENTED_EDGE('',*,*,#22902,.T.);
#30517=ORIENTED_EDGE('',*,*,#22903,.F.);
#30518=ORIENTED_EDGE('',*,*,#22904,.F.);
#30519=ORIENTED_EDGE('',*,*,#22905,.F.);
#30520=ORIENTED_EDGE('',*,*,#22906,.T.);
#30521=ORIENTED_EDGE('',*,*,#22895,.T.);
#30522=ORIENTED_EDGE('',*,*,#22907,.F.);
#30523=ORIENTED_EDGE('',*,*,#22908,.F.);
#30524=ORIENTED_EDGE('',*,*,#22909,.T.);
#30525=ORIENTED_EDGE('',*,*,#22894,.T.);
#30526=ORIENTED_EDGE('',*,*,#22910,.F.);
#30527=ORIENTED_EDGE('',*,*,#22911,.F.);
#30528=ORIENTED_EDGE('',*,*,#22907,.T.);
#30529=ORIENTED_EDGE('',*,*,#22893,.F.);
#30530=ORIENTED_EDGE('',*,*,#22912,.F.);
#30531=ORIENTED_EDGE('',*,*,#22913,.T.);
#30532=ORIENTED_EDGE('',*,*,#22910,.T.);
#30533=ORIENTED_EDGE('',*,*,#22896,.F.);
#30534=ORIENTED_EDGE('',*,*,#22909,.F.);
#30535=ORIENTED_EDGE('',*,*,#22914,.T.);
#30536=ORIENTED_EDGE('',*,*,#22912,.T.);
#30537=ORIENTED_EDGE('',*,*,#22908,.T.);
#30538=ORIENTED_EDGE('',*,*,#22911,.T.);
#30539=ORIENTED_EDGE('',*,*,#22913,.F.);
#30540=ORIENTED_EDGE('',*,*,#22914,.F.);
#30541=ORIENTED_EDGE('',*,*,#22915,.F.);
#30542=ORIENTED_EDGE('',*,*,#22916,.F.);
#30543=ORIENTED_EDGE('',*,*,#22917,.F.);
#30544=ORIENTED_EDGE('',*,*,#22918,.F.);
#30545=ORIENTED_EDGE('',*,*,#22905,.T.);
#30546=ORIENTED_EDGE('',*,*,#22919,.F.);
#30547=ORIENTED_EDGE('',*,*,#22920,.F.);
#30548=ORIENTED_EDGE('',*,*,#22904,.T.);
#30549=ORIENTED_EDGE('',*,*,#22921,.T.);
#30550=ORIENTED_EDGE('',*,*,#22922,.T.);
#30551=ORIENTED_EDGE('',*,*,#22923,.T.);
#30552=ORIENTED_EDGE('',*,*,#22903,.T.);
#30553=ORIENTED_EDGE('',*,*,#22924,.T.);
#30554=ORIENTED_EDGE('',*,*,#22925,.T.);
#30555=ORIENTED_EDGE('',*,*,#22926,.F.);
#30556=ORIENTED_EDGE('',*,*,#22881,.F.);
#30557=ORIENTED_EDGE('',*,*,#22927,.T.);
#30558=ORIENTED_EDGE('',*,*,#22928,.F.);
#30559=ORIENTED_EDGE('',*,*,#22929,.F.);
#30560=ORIENTED_EDGE('',*,*,#22906,.F.);
#30561=ORIENTED_EDGE('',*,*,#22930,.F.);
#30562=ORIENTED_EDGE('',*,*,#22931,.F.);
#30563=ORIENTED_EDGE('',*,*,#22932,.T.);
#30564=ORIENTED_EDGE('',*,*,#22926,.T.);
#30565=ORIENTED_EDGE('',*,*,#22933,.F.);
#30566=ORIENTED_EDGE('',*,*,#22934,.F.);
#30567=ORIENTED_EDGE('',*,*,#22882,.F.);
#30568=ORIENTED_EDGE('',*,*,#22900,.T.);
#30569=ORIENTED_EDGE('',*,*,#22935,.F.);
#30570=ORIENTED_EDGE('',*,*,#22936,.F.);
#30571=ORIENTED_EDGE('',*,*,#22899,.T.);
#30572=ORIENTED_EDGE('',*,*,#22937,.T.);
#30573=ORIENTED_EDGE('',*,*,#22938,.T.);
#30574=ORIENTED_EDGE('',*,*,#22939,.T.);
#30575=ORIENTED_EDGE('',*,*,#22898,.T.);
#30576=ORIENTED_EDGE('',*,*,#22940,.T.);
#30577=ORIENTED_EDGE('',*,*,#22941,.T.);
#30578=ORIENTED_EDGE('',*,*,#22942,.F.);
#30579=ORIENTED_EDGE('',*,*,#22883,.F.);
#30580=ORIENTED_EDGE('',*,*,#22934,.T.);
#30581=ORIENTED_EDGE('',*,*,#22943,.F.);
#30582=ORIENTED_EDGE('',*,*,#22944,.F.);
#30583=ORIENTED_EDGE('',*,*,#22901,.F.);
#30584=ORIENTED_EDGE('',*,*,#22945,.F.);
#30585=ORIENTED_EDGE('',*,*,#22946,.F.);
#30586=ORIENTED_EDGE('',*,*,#22947,.T.);
#30587=ORIENTED_EDGE('',*,*,#22942,.T.);
#30588=ORIENTED_EDGE('',*,*,#22948,.T.);
#30589=ORIENTED_EDGE('',*,*,#22927,.F.);
#30590=ORIENTED_EDGE('',*,*,#22884,.F.);
#30591=ORIENTED_EDGE('',*,*,#22887,.F.);
#30592=ORIENTED_EDGE('',*,*,#22847,.F.);
#30593=ORIENTED_EDGE('',*,*,#22949,.T.);
#30594=ORIENTED_EDGE('',*,*,#22852,.T.);
#30595=ORIENTED_EDGE('',*,*,#22950,.F.);
#30596=ORIENTED_EDGE('',*,*,#22855,.T.);
#30597=ORIENTED_EDGE('',*,*,#22886,.T.);
#30598=ORIENTED_EDGE('',*,*,#22951,.F.);
#30599=ORIENTED_EDGE('',*,*,#22861,.F.);
#30600=ORIENTED_EDGE('',*,*,#22952,.T.);
#30601=ORIENTED_EDGE('',*,*,#22953,.T.);
#30602=ORIENTED_EDGE('',*,*,#22888,.F.);
#30603=ORIENTED_EDGE('',*,*,#22949,.F.);
#30604=ORIENTED_EDGE('',*,*,#22846,.T.);
#30605=ORIENTED_EDGE('',*,*,#22954,.T.);
#30606=ORIENTED_EDGE('',*,*,#22955,.F.);
#30607=ORIENTED_EDGE('',*,*,#22956,.F.);
#30608=ORIENTED_EDGE('',*,*,#22950,.T.);
#30609=ORIENTED_EDGE('',*,*,#22957,.T.);
#30610=ORIENTED_EDGE('',*,*,#22952,.F.);
#30611=ORIENTED_EDGE('',*,*,#22958,.F.);
#30612=ORIENTED_EDGE('',*,*,#22959,.T.);
#30613=ORIENTED_EDGE('',*,*,#22960,.T.);
#30614=ORIENTED_EDGE('',*,*,#22849,.F.);
#30615=ORIENTED_EDGE('',*,*,#22885,.T.);
#30616=ORIENTED_EDGE('',*,*,#22953,.F.);
#30617=ORIENTED_EDGE('',*,*,#22957,.F.);
#30618=ORIENTED_EDGE('',*,*,#22951,.T.);
#30619=ORIENTED_EDGE('',*,*,#22891,.F.);
#30620=ORIENTED_EDGE('',*,*,#22869,.F.);
#30621=ORIENTED_EDGE('',*,*,#22961,.T.);
#30622=ORIENTED_EDGE('',*,*,#22866,.T.);
#30623=ORIENTED_EDGE('',*,*,#22962,.F.);
#30624=ORIENTED_EDGE('',*,*,#22878,.T.);
#30625=ORIENTED_EDGE('',*,*,#22890,.T.);
#30626=ORIENTED_EDGE('',*,*,#22963,.F.);
#30627=ORIENTED_EDGE('',*,*,#22874,.F.);
#30628=ORIENTED_EDGE('',*,*,#22964,.T.);
#30629=ORIENTED_EDGE('',*,*,#22965,.T.);
#30630=ORIENTED_EDGE('',*,*,#22892,.F.);
#30631=ORIENTED_EDGE('',*,*,#22863,.F.);
#30632=ORIENTED_EDGE('',*,*,#22961,.F.);
#30633=ORIENTED_EDGE('',*,*,#22868,.T.);
#30634=ORIENTED_EDGE('',*,*,#22966,.T.);
#30635=ORIENTED_EDGE('',*,*,#22967,.F.);
#30636=ORIENTED_EDGE('',*,*,#22968,.F.);
#30637=ORIENTED_EDGE('',*,*,#22962,.T.);
#30638=ORIENTED_EDGE('',*,*,#22969,.T.);
#30639=ORIENTED_EDGE('',*,*,#22964,.F.);
#30640=ORIENTED_EDGE('',*,*,#22970,.F.);
#30641=ORIENTED_EDGE('',*,*,#22971,.T.);
#30642=ORIENTED_EDGE('',*,*,#22972,.T.);
#30643=ORIENTED_EDGE('',*,*,#22889,.T.);
#30644=ORIENTED_EDGE('',*,*,#22965,.F.);
#30645=ORIENTED_EDGE('',*,*,#22969,.F.);
#30646=ORIENTED_EDGE('',*,*,#22963,.T.);
#30647=ORIENTED_EDGE('',*,*,#22973,.F.);
#30648=ORIENTED_EDGE('',*,*,#22954,.F.);
#30649=ORIENTED_EDGE('',*,*,#22853,.F.);
#30650=ORIENTED_EDGE('',*,*,#22974,.F.);
#30651=ORIENTED_EDGE('',*,*,#22975,.T.);
#30652=ORIENTED_EDGE('',*,*,#22976,.F.);
#30653=ORIENTED_EDGE('',*,*,#22858,.T.);
#30654=ORIENTED_EDGE('',*,*,#22960,.F.);
#30655=ORIENTED_EDGE('',*,*,#22837,.F.);
#30656=ORIENTED_EDGE('',*,*,#22956,.T.);
#30657=ORIENTED_EDGE('',*,*,#22977,.T.);
#30658=ORIENTED_EDGE('',*,*,#22958,.T.);
#30659=ORIENTED_EDGE('',*,*,#22860,.F.);
#30660=ORIENTED_EDGE('',*,*,#22978,.T.);
#30661=ORIENTED_EDGE('',*,*,#22979,.F.);
#30662=ORIENTED_EDGE('',*,*,#22980,.T.);
#30663=ORIENTED_EDGE('',*,*,#22856,.T.);
#30664=ORIENTED_EDGE('',*,*,#22835,.T.);
#30665=ORIENTED_EDGE('',*,*,#22981,.F.);
#30666=ORIENTED_EDGE('',*,*,#22975,.F.);
#30667=ORIENTED_EDGE('',*,*,#22982,.T.);
#30668=ORIENTED_EDGE('',*,*,#22979,.T.);
#30669=ORIENTED_EDGE('',*,*,#22983,.F.);
#30670=ORIENTED_EDGE('',*,*,#22966,.F.);
#30671=ORIENTED_EDGE('',*,*,#22876,.F.);
#30672=ORIENTED_EDGE('',*,*,#22984,.F.);
#30673=ORIENTED_EDGE('',*,*,#22985,.T.);
#30674=ORIENTED_EDGE('',*,*,#22986,.F.);
#30675=ORIENTED_EDGE('',*,*,#22871,.T.);
#30676=ORIENTED_EDGE('',*,*,#22972,.F.);
#30677=ORIENTED_EDGE('',*,*,#22840,.F.);
#30678=ORIENTED_EDGE('',*,*,#22968,.T.);
#30679=ORIENTED_EDGE('',*,*,#22987,.T.);
#30680=ORIENTED_EDGE('',*,*,#22970,.T.);
#30681=ORIENTED_EDGE('',*,*,#22873,.F.);
#30682=ORIENTED_EDGE('',*,*,#22988,.F.);
#30683=ORIENTED_EDGE('',*,*,#22989,.F.);
#30684=ORIENTED_EDGE('',*,*,#22990,.F.);
#30685=ORIENTED_EDGE('',*,*,#22879,.T.);
#30686=ORIENTED_EDGE('',*,*,#22838,.T.);
#30687=ORIENTED_EDGE('',*,*,#22991,.F.);
#30688=ORIENTED_EDGE('',*,*,#22985,.F.);
#30689=ORIENTED_EDGE('',*,*,#22992,.F.);
#30690=ORIENTED_EDGE('',*,*,#22989,.T.);
#30691=ORIENTED_EDGE('',*,*,#22984,.T.);
#30692=ORIENTED_EDGE('',*,*,#22880,.T.);
#30693=ORIENTED_EDGE('',*,*,#22990,.T.);
#30694=ORIENTED_EDGE('',*,*,#22992,.T.);
#30695=ORIENTED_EDGE('',*,*,#22986,.T.);
#30696=ORIENTED_EDGE('',*,*,#22991,.T.);
#30697=ORIENTED_EDGE('',*,*,#22988,.T.);
#30698=ORIENTED_EDGE('',*,*,#22872,.F.);
#30699=ORIENTED_EDGE('',*,*,#22974,.T.);
#30700=ORIENTED_EDGE('',*,*,#22857,.T.);
#30701=ORIENTED_EDGE('',*,*,#22980,.F.);
#30702=ORIENTED_EDGE('',*,*,#22982,.F.);
#30703=ORIENTED_EDGE('',*,*,#22976,.T.);
#30704=ORIENTED_EDGE('',*,*,#22981,.T.);
#30705=ORIENTED_EDGE('',*,*,#22978,.F.);
#30706=ORIENTED_EDGE('',*,*,#22859,.F.);
#30707=ORIENTED_EDGE('',*,*,#22983,.T.);
#30708=ORIENTED_EDGE('',*,*,#22971,.F.);
#30709=ORIENTED_EDGE('',*,*,#22987,.F.);
#30710=ORIENTED_EDGE('',*,*,#22967,.T.);
#30711=ORIENTED_EDGE('',*,*,#22955,.T.);
#30712=ORIENTED_EDGE('',*,*,#22973,.T.);
#30713=ORIENTED_EDGE('',*,*,#22959,.F.);
#30714=ORIENTED_EDGE('',*,*,#22977,.F.);
#30715=ORIENTED_EDGE('',*,*,#22993,.F.);
#30716=ORIENTED_EDGE('',*,*,#22937,.F.);
#30717=ORIENTED_EDGE('',*,*,#22994,.T.);
#30718=ORIENTED_EDGE('',*,*,#22932,.F.);
#30719=ORIENTED_EDGE('',*,*,#22995,.F.);
#30720=ORIENTED_EDGE('',*,*,#22947,.F.);
#30721=ORIENTED_EDGE('',*,*,#22996,.T.);
#30722=ORIENTED_EDGE('',*,*,#22921,.F.);
#30723=ORIENTED_EDGE('',*,*,#22923,.F.);
#30724=ORIENTED_EDGE('',*,*,#22997,.F.);
#30725=ORIENTED_EDGE('',*,*,#22945,.T.);
#30726=ORIENTED_EDGE('',*,*,#22995,.T.);
#30727=ORIENTED_EDGE('',*,*,#22922,.F.);
#30728=ORIENTED_EDGE('',*,*,#22996,.F.);
#30729=ORIENTED_EDGE('',*,*,#22946,.T.);
#30730=ORIENTED_EDGE('',*,*,#22997,.T.);
#30731=ORIENTED_EDGE('',*,*,#22925,.F.);
#30732=ORIENTED_EDGE('',*,*,#22998,.F.);
#30733=ORIENTED_EDGE('',*,*,#22943,.T.);
#30734=ORIENTED_EDGE('',*,*,#22933,.T.);
#30735=ORIENTED_EDGE('',*,*,#22924,.F.);
#30736=ORIENTED_EDGE('',*,*,#22902,.F.);
#30737=ORIENTED_EDGE('',*,*,#22944,.T.);
#30738=ORIENTED_EDGE('',*,*,#22998,.T.);
#30739=ORIENTED_EDGE('',*,*,#22929,.T.);
#30740=ORIENTED_EDGE('',*,*,#22999,.F.);
#30741=ORIENTED_EDGE('',*,*,#22940,.F.);
#30742=ORIENTED_EDGE('',*,*,#22897,.T.);
#30743=ORIENTED_EDGE('',*,*,#22928,.T.);
#30744=ORIENTED_EDGE('',*,*,#22948,.F.);
#30745=ORIENTED_EDGE('',*,*,#22941,.F.);
#30746=ORIENTED_EDGE('',*,*,#22999,.T.);
#30747=ORIENTED_EDGE('',*,*,#22931,.T.);
#30748=ORIENTED_EDGE('',*,*,#23000,.F.);
#30749=ORIENTED_EDGE('',*,*,#22938,.F.);
#30750=ORIENTED_EDGE('',*,*,#22993,.T.);
#30751=ORIENTED_EDGE('',*,*,#22930,.T.);
#30752=ORIENTED_EDGE('',*,*,#22994,.F.);
#30753=ORIENTED_EDGE('',*,*,#22939,.F.);
#30754=ORIENTED_EDGE('',*,*,#23000,.T.);
#30755=ORIENTED_EDGE('',*,*,#22917,.T.);
#30756=ORIENTED_EDGE('',*,*,#23001,.F.);
#30757=ORIENTED_EDGE('',*,*,#22842,.F.);
#30758=ORIENTED_EDGE('',*,*,#23002,.T.);
#30759=ORIENTED_EDGE('',*,*,#22916,.T.);
#30760=ORIENTED_EDGE('',*,*,#23003,.F.);
#30761=ORIENTED_EDGE('',*,*,#22843,.F.);
#30762=ORIENTED_EDGE('',*,*,#23001,.T.);
#30763=ORIENTED_EDGE('',*,*,#22915,.T.);
#30764=ORIENTED_EDGE('',*,*,#23004,.F.);
#30765=ORIENTED_EDGE('',*,*,#22844,.F.);
#30766=ORIENTED_EDGE('',*,*,#23003,.T.);
#30767=ORIENTED_EDGE('',*,*,#22918,.T.);
#30768=ORIENTED_EDGE('',*,*,#23002,.F.);
#30769=ORIENTED_EDGE('',*,*,#22841,.T.);
#30770=ORIENTED_EDGE('',*,*,#23004,.T.);
#30771=ORIENTED_EDGE('',*,*,#22920,.T.);
#30772=ORIENTED_EDGE('',*,*,#23005,.T.);
#30773=ORIENTED_EDGE('',*,*,#23005,.F.);
#30774=ORIENTED_EDGE('',*,*,#22919,.T.);
#30775=ORIENTED_EDGE('',*,*,#22936,.T.);
#30776=ORIENTED_EDGE('',*,*,#23006,.T.);
#30777=ORIENTED_EDGE('',*,*,#23006,.F.);
#30778=ORIENTED_EDGE('',*,*,#22935,.T.);
#38002=CYLINDRICAL_SURFACE('',#41231,1.);
#38003=CYLINDRICAL_SURFACE('',#41234,1.);
#38004=CYLINDRICAL_SURFACE('',#41237,56.);
#38005=CYLINDRICAL_SURFACE('',#41287,1.);
#38006=CYLINDRICAL_SURFACE('',#41288,1.);
#38699=ADVANCED_FACE('',(#3011),#970,.F.);
#38700=ADVANCED_FACE('',(#3012),#971,.F.);
#38701=ADVANCED_FACE('',(#3013),#972,.F.);
#38702=ADVANCED_FACE('',(#3014),#973,.F.);
#38703=ADVANCED_FACE('',(#3015),#974,.F.);
#38704=ADVANCED_FACE('',(#3016),#975,.F.);
#38705=ADVANCED_FACE('',(#3017),#38002,.F.);
#38706=ADVANCED_FACE('',(#3018),#38003,.F.);
#38707=ADVANCED_FACE('',(#3019),#38004,.F.);
#38708=ADVANCED_FACE('',(#3020),#976,.F.);
#38709=ADVANCED_FACE('',(#3021),#977,.T.);
#38710=ADVANCED_FACE('',(#3022),#978,.F.);
#38711=ADVANCED_FACE('',(#3023),#979,.T.);
#38712=ADVANCED_FACE('',(#3024),#980,.T.);
#38713=ADVANCED_FACE('',(#3025),#981,.F.);
#38714=ADVANCED_FACE('',(#3026),#982,.T.);
#38715=ADVANCED_FACE('',(#3027),#983,.F.);
#38716=ADVANCED_FACE('',(#3028,#247,#248),#984,.T.);
#38717=ADVANCED_FACE('',(#3029,#249),#985,.F.);
#38718=ADVANCED_FACE('',(#3030),#986,.F.);
#38719=ADVANCED_FACE('',(#3031),#987,.F.);
#38720=ADVANCED_FACE('',(#3032),#988,.T.);
#38721=ADVANCED_FACE('',(#3033),#989,.T.);
#38722=ADVANCED_FACE('',(#3034,#250),#990,.T.);
#38723=ADVANCED_FACE('',(#3035),#991,.F.);
#38724=ADVANCED_FACE('',(#3036),#992,.F.);
#38725=ADVANCED_FACE('',(#3037),#993,.F.);
#38726=ADVANCED_FACE('',(#3038),#994,.F.);
#38727=ADVANCED_FACE('',(#3039),#995,.T.);
#38728=ADVANCED_FACE('',(#3040),#996,.F.);
#38729=ADVANCED_FACE('',(#3041),#997,.T.);
#38730=ADVANCED_FACE('',(#3042),#998,.F.);
#38731=ADVANCED_FACE('',(#3043),#999,.F.);
#38732=ADVANCED_FACE('',(#3044),#1000,.T.);
#38733=ADVANCED_FACE('',(#3045),#1001,.F.);
#38734=ADVANCED_FACE('',(#3046),#1002,.T.);
#38735=ADVANCED_FACE('',(#3047),#1003,.F.);
#38736=ADVANCED_FACE('',(#3048),#1004,.F.);
#38737=ADVANCED_FACE('',(#3049,#251),#1005,.T.);
#38738=ADVANCED_FACE('',(#3050,#252),#1006,.F.);
#38739=ADVANCED_FACE('',(#3051),#1007,.T.);
#38740=ADVANCED_FACE('',(#3052,#253),#1008,.T.);
#38741=ADVANCED_FACE('',(#3053,#254),#1009,.F.);
#38742=ADVANCED_FACE('',(#3054),#1010,.T.);
#38743=ADVANCED_FACE('',(#3055),#1011,.F.);
#38744=ADVANCED_FACE('',(#3056),#1012,.F.);
#38745=ADVANCED_FACE('',(#3057),#1013,.F.);
#38746=ADVANCED_FACE('',(#3058),#1014,.F.);
#38747=ADVANCED_FACE('',(#3059),#38005,.F.);
#38748=ADVANCED_FACE('',(#3060),#38006,.F.);
#38749=ADVANCED_FACE('',(#3061),#1015,.F.);
#38750=ADVANCED_FACE('',(#3062),#1016,.F.);
#38751=ADVANCED_FACE('',(#3063),#1017,.T.);
#38752=ADVANCED_FACE('',(#3064),#1018,.T.);
#38753=ADVANCED_FACE('',(#3065),#1019,.T.);
#38754=ADVANCED_FACE('',(#3066),#1020,.T.);
#38755=ADVANCED_FACE('',(#3067),#1021,.F.);
#38756=ADVANCED_FACE('',(#3068),#1022,.F.);
#38757=ADVANCED_FACE('',(#3069),#1023,.F.);
#38758=ADVANCED_FACE('',(#3070),#1024,.F.);
#38759=ADVANCED_FACE('',(#3071),#1025,.F.);
#38760=ADVANCED_FACE('',(#3072),#1026,.F.);
#38761=ADVANCED_FACE('',(#3073),#1027,.F.);
#38762=ADVANCED_FACE('',(#3074),#1028,.F.);
#38763=ADVANCED_FACE('',(#3075),#27,.T.);
#38764=ADVANCED_FACE('',(#3076),#28,.T.);
#39935=CLOSED_SHELL('',(#38699,#38700,#38701,#38702,#38703,#38704));
#39936=CLOSED_SHELL('',(#38705,#38706,#38707,#38708,#38709,#38710,#38711,
#38712,#38713,#38714,#38715,#38716,#38717,#38718,#38719,#38720,#38721,#38722,
#38723,#38724,#38725,#38726,#38727,#38728,#38729,#38730,#38731,#38732,#38733,
#38734,#38735,#38736,#38737,#38738,#38739,#38740,#38741,#38742,#38743,#38744,
#38745,#38746,#38747,#38748,#38749,#38750,#38751,#38752,#38753,#38754,#38755,
#38756,#38757,#38758,#38759,#38760,#38761,#38762,#38763,#38764));
#41224=AXIS2_PLACEMENT_3D('',#57979,#46267,#46268);
#41225=AXIS2_PLACEMENT_3D('',#57980,#46269,#46270);
#41226=AXIS2_PLACEMENT_3D('',#57989,#46275,#46276);
#41227=AXIS2_PLACEMENT_3D('',#57998,#46281,#46282);
#41228=AXIS2_PLACEMENT_3D('',#58001,#46285,#46286);
#41229=AXIS2_PLACEMENT_3D('',#58003,#46288,#46289);
#41230=AXIS2_PLACEMENT_3D('',#58005,#46291,#46292);
#41231=AXIS2_PLACEMENT_3D('',#58006,#46293,#46294);
#41232=AXIS2_PLACEMENT_3D('',#58008,#46295,#46296);
#41233=AXIS2_PLACEMENT_3D('',#58011,#46298,#46299);
#41234=AXIS2_PLACEMENT_3D('',#58012,#46300,#46301);
#41235=AXIS2_PLACEMENT_3D('',#58014,#46302,#46303);
#41236=AXIS2_PLACEMENT_3D('',#58017,#46305,#46306);
#41237=AXIS2_PLACEMENT_3D('',#58018,#46307,#46308);
#41238=AXIS2_PLACEMENT_3D('',#58021,#46309,#46310);
#41239=AXIS2_PLACEMENT_3D('',#58025,#46312,#46313);
#41240=AXIS2_PLACEMENT_3D('',#58027,#46315,#46316);
#41241=AXIS2_PLACEMENT_3D('',#58036,#46321,#46322);
#41242=AXIS2_PLACEMENT_3D('',#58045,#46327,#46328);
#41243=AXIS2_PLACEMENT_3D('',#58055,#46334,#46335);
#41244=AXIS2_PLACEMENT_3D('',#58065,#46341,#46342);
#41245=AXIS2_PLACEMENT_3D('',#58074,#46347,#46348);
#41246=AXIS2_PLACEMENT_3D('',#58083,#46353,#46354);
#41247=AXIS2_PLACEMENT_3D('',#58093,#46360,#46361);
#41248=AXIS2_PLACEMENT_3D('',#58103,#46367,#46368);
#41249=AXIS2_PLACEMENT_3D('',#58124,#46381,#46382);
#41250=AXIS2_PLACEMENT_3D('',#58153,#46397,#46398);
#41251=AXIS2_PLACEMENT_3D('',#58159,#46402,#46403);
#41252=AXIS2_PLACEMENT_3D('',#58163,#46406,#46407);
#41253=AXIS2_PLACEMENT_3D('',#58167,#46410,#46411);
#41254=AXIS2_PLACEMENT_3D('',#58169,#46413,#46414);
#41255=AXIS2_PLACEMENT_3D('',#58178,#46419,#46420);
#41256=AXIS2_PLACEMENT_3D('',#58180,#46421,#46422);
#41257=AXIS2_PLACEMENT_3D('',#58181,#46423,#46424);
#41258=AXIS2_PLACEMENT_3D('',#58202,#46437,#46438);
#41259=AXIS2_PLACEMENT_3D('',#58206,#46441,#46442);
#41260=AXIS2_PLACEMENT_3D('',#58208,#46443,#46444);
#41261=AXIS2_PLACEMENT_3D('',#58209,#46445,#46446);
#41262=AXIS2_PLACEMENT_3D('',#58228,#46458,#46459);
#41263=AXIS2_PLACEMENT_3D('',#58230,#46461,#46462);
#41264=AXIS2_PLACEMENT_3D('',#58232,#46464,#46465);
#41265=AXIS2_PLACEMENT_3D('',#58236,#46468,#46469);
#41266=AXIS2_PLACEMENT_3D('',#58240,#46472,#46473);
#41267=AXIS2_PLACEMENT_3D('',#58252,#46481,#46482);
#41268=AXIS2_PLACEMENT_3D('',#58253,#46483,#46484);
#41269=AXIS2_PLACEMENT_3D('',#58255,#46486,#46487);
#41270=AXIS2_PLACEMENT_3D('',#58259,#46490,#46491);
#41271=AXIS2_PLACEMENT_3D('',#58263,#46494,#46495);
#41272=AXIS2_PLACEMENT_3D('',#58275,#46503,#46504);
#41273=AXIS2_PLACEMENT_3D('',#58276,#46505,#46506);
#41274=AXIS2_PLACEMENT_3D('',#58277,#46507,#46508);
#41275=AXIS2_PLACEMENT_3D('',#58283,#46512,#46513);
#41276=AXIS2_PLACEMENT_3D('',#58284,#46514,#46515);
#41277=AXIS2_PLACEMENT_3D('',#58290,#46519,#46520);
#41278=AXIS2_PLACEMENT_3D('',#58293,#46523,#46524);
#41279=AXIS2_PLACEMENT_3D('',#58294,#46525,#46526);
#41280=AXIS2_PLACEMENT_3D('',#58300,#46530,#46531);
#41281=AXIS2_PLACEMENT_3D('',#58301,#46532,#46533);
#41282=AXIS2_PLACEMENT_3D('',#58307,#46537,#46538);
#41283=AXIS2_PLACEMENT_3D('',#58310,#46541,#46542);
#41284=AXIS2_PLACEMENT_3D('',#58311,#46543,#46544);
#41285=AXIS2_PLACEMENT_3D('',#58312,#46545,#46546);
#41286=AXIS2_PLACEMENT_3D('',#58313,#46547,#46548);
#41287=AXIS2_PLACEMENT_3D('',#58314,#46549,#46550);
#41288=AXIS2_PLACEMENT_3D('',#58315,#46551,#46552);
#41289=AXIS2_PLACEMENT_3D('',#58316,#46553,#46554);
#41290=AXIS2_PLACEMENT_3D('',#58319,#46557,#46558);
#41291=AXIS2_PLACEMENT_3D('',#58322,#46561,#46562);
#41292=AXIS2_PLACEMENT_3D('',#58324,#46564,#46565);
#41293=AXIS2_PLACEMENT_3D('',#58325,#46566,#46567);
#41294=AXIS2_PLACEMENT_3D('',#58327,#46569,#46570);
#41295=AXIS2_PLACEMENT_3D('',#58328,#46571,#46572);
#41296=AXIS2_PLACEMENT_3D('',#58330,#46574,#46575);
#41297=AXIS2_PLACEMENT_3D('',#58331,#46576,#46577);
#41298=AXIS2_PLACEMENT_3D('',#58333,#46579,#46580);
#41299=AXIS2_PLACEMENT_3D('',#58334,#46581,#46582);
#41300=AXIS2_PLACEMENT_3D('',#58337,#46585,#46586);
#41301=AXIS2_PLACEMENT_3D('',#58339,#46588,#46589);
#41302=AXIS2_PLACEMENT_3D('',#58341,#46591,#46592);
#41303=AXIS2_PLACEMENT_3D('',#58342,#46593,#46594);
#41304=AXIS2_PLACEMENT_3D('',#58344,#46595,#46596);
#41305=AXIS2_PLACEMENT_3D('',#58345,#46597,#46598);
#41306=AXIS2_PLACEMENT_3D('',#58347,#46599,#46600);
#46267=DIRECTION('axis',(0.,0.,1.));
#46268=DIRECTION('refdir',(1.,0.,0.));
#46269=DIRECTION('center_axis',(0.,0.,1.));
#46270=DIRECTION('ref_axis',(1.,0.,0.));
#46271=DIRECTION('',(0.,-1.,0.));
#46272=DIRECTION('',(-1.,0.,0.));
#46273=DIRECTION('',(0.,1.,0.));
#46274=DIRECTION('',(1.,0.,0.));
#46275=DIRECTION('center_axis',(0.,0.,-1.));
#46276=DIRECTION('ref_axis',(-1.,0.,0.));
#46277=DIRECTION('',(1.,-6.42490176287706E-17,0.));
#46278=DIRECTION('',(0.,1.,0.));
#46279=DIRECTION('',(-1.,0.,0.));
#46280=DIRECTION('',(0.,-1.,0.));
#46281=DIRECTION('center_axis',(-6.42490176287706E-17,-1.,0.));
#46282=DIRECTION('ref_axis',(1.,-6.42490176287706E-17,0.));
#46283=DIRECTION('',(0.,0.,1.));
#46284=DIRECTION('',(0.,0.,1.));
#46285=DIRECTION('center_axis',(-1.,0.,0.));
#46286=DIRECTION('ref_axis',(0.,0.,1.));
#46287=DIRECTION('',(0.,0.,1.));
#46288=DIRECTION('center_axis',(0.,1.,0.));
#46289=DIRECTION('ref_axis',(0.,0.,1.));
#46290=DIRECTION('',(0.,0.,1.));
#46291=DIRECTION('center_axis',(1.,0.,0.));
#46292=DIRECTION('ref_axis',(0.,0.,-1.));
#46293=DIRECTION('center_axis',(1.,-3.61400724161835E-16,0.));
#46294=DIRECTION('ref_axis',(3.61400724161835E-16,1.,0.));
#46295=DIRECTION('center_axis',(1.,-4.33680868994202E-17,0.));
#46296=DIRECTION('ref_axis',(4.33680868994202E-17,1.,0.));
#46297=DIRECTION('',(1.,-3.61400724161835E-16,0.));
#46298=DIRECTION('center_axis',(1.,-3.61400724161835E-16,0.));
#46299=DIRECTION('ref_axis',(3.61400724161835E-16,1.,0.));
#46300=DIRECTION('center_axis',(1.,-3.61400724161835E-16,0.));
#46301=DIRECTION('ref_axis',(3.61400724161835E-16,1.,0.));
#46302=DIRECTION('center_axis',(1.,0.,0.));
#46303=DIRECTION('ref_axis',(0.,0.,-1.));
#46304=DIRECTION('',(1.,-3.61400724161835E-16,0.));
#46305=DIRECTION('center_axis',(1.,-3.46944695195361E-16,0.));
#46306=DIRECTION('ref_axis',(3.46944695195361E-16,1.,0.));
#46307=DIRECTION('center_axis',(0.,-1.,0.));
#46308=DIRECTION('ref_axis',(0.,0.,-1.));
#46309=DIRECTION('center_axis',(0.,-1.,0.));
#46310=DIRECTION('ref_axis',(0.,0.,-1.));
#46311=DIRECTION('',(0.,-1.,0.));
#46312=DIRECTION('center_axis',(0.,-1.,0.));
#46313=DIRECTION('ref_axis',(0.,0.,-1.));
#46314=DIRECTION('',(0.,1.,0.));
#46315=DIRECTION('center_axis',(0.,1.,0.));
#46316=DIRECTION('ref_axis',(0.,0.,1.));
#46317=DIRECTION('',(0.,0.,1.));
#46318=DIRECTION('',(-1.,0.,0.));
#46319=DIRECTION('',(0.,0.,1.));
#46320=DIRECTION('',(-1.,0.,0.));
#46321=DIRECTION('center_axis',(0.,1.,0.));
#46322=DIRECTION('ref_axis',(0.,0.,1.));
#46323=DIRECTION('',(-1.,0.,0.));
#46324=DIRECTION('',(0.,0.,1.));
#46325=DIRECTION('',(-1.,0.,0.));
#46326=DIRECTION('',(0.,0.,1.));
#46327=DIRECTION('center_axis',(0.,1.,0.));
#46328=DIRECTION('ref_axis',(0.,0.,1.));
#46329=DIRECTION('',(0.,0.,1.));
#46330=DIRECTION('',(-1.,0.,0.));
#46331=DIRECTION('',(4.33680868994201E-16,0.,1.));
#46332=DIRECTION('',(0.,0.,1.));
#46333=DIRECTION('',(-1.,0.,0.));
#46334=DIRECTION('center_axis',(0.,1.,0.));
#46335=DIRECTION('ref_axis',(0.,0.,1.));
#46336=DIRECTION('',(0.,0.,1.));
#46337=DIRECTION('',(-1.,0.,0.));
#46338=DIRECTION('',(0.,0.,1.));
#46339=DIRECTION('',(4.33680868994201E-16,0.,1.));
#46340=DIRECTION('',(-1.,0.,0.));
#46341=DIRECTION('center_axis',(0.,1.,0.));
#46342=DIRECTION('ref_axis',(0.,0.,1.));
#46343=DIRECTION('',(-1.,0.,0.));
#46344=DIRECTION('',(0.,0.,1.));
#46345=DIRECTION('',(-1.,0.,0.));
#46346=DIRECTION('',(0.,0.,1.));
#46347=DIRECTION('center_axis',(0.,1.,0.));
#46348=DIRECTION('ref_axis',(0.,0.,1.));
#46349=DIRECTION('',(0.,0.,1.));
#46350=DIRECTION('',(-1.,0.,0.));
#46351=DIRECTION('',(0.,0.,1.));
#46352=DIRECTION('',(-1.,0.,0.));
#46353=DIRECTION('center_axis',(0.,1.,0.));
#46354=DIRECTION('ref_axis',(0.,0.,1.));
#46355=DIRECTION('',(0.,0.,1.));
#46356=DIRECTION('',(-1.,0.,0.));
#46357=DIRECTION('',(0.,0.,1.));
#46358=DIRECTION('',(0.,0.,1.));
#46359=DIRECTION('',(-1.,0.,0.));
#46360=DIRECTION('center_axis',(0.,1.,0.));
#46361=DIRECTION('ref_axis',(0.,0.,1.));
#46362=DIRECTION('',(0.,0.,1.));
#46363=DIRECTION('',(-1.,0.,0.));
#46364=DIRECTION('',(0.,0.,1.));
#46365=DIRECTION('',(0.,0.,1.));
#46366=DIRECTION('',(-1.,0.,0.));
#46367=DIRECTION('center_axis',(0.,0.,-1.));
#46368=DIRECTION('ref_axis',(-1.,0.,0.));
#46369=DIRECTION('',(-1.,6.08674903851511E-17,0.));
#46370=DIRECTION('',(0.,1.,0.));
#46371=DIRECTION('',(1.,0.,0.));
#46372=DIRECTION('',(0.,-1.,0.));
#46373=DIRECTION('',(0.,1.,0.));
#46374=DIRECTION('',(-1.,0.,0.));
#46375=DIRECTION('',(0.,1.,0.));
#46376=DIRECTION('',(-1.,0.,0.));
#46377=DIRECTION('',(0.,1.,0.));
#46378=DIRECTION('',(-1.,0.,0.));
#46379=DIRECTION('',(0.,1.,0.));
#46380=DIRECTION('',(-1.,0.,0.));
#46381=DIRECTION('center_axis',(0.,0.,1.));
#46382=DIRECTION('ref_axis',(1.,0.,0.));
#46383=DIRECTION('',(1.,5.9818050895752E-17,0.));
#46384=DIRECTION('',(8.46206573647223E-17,1.,0.));
#46385=DIRECTION('',(1.,0.,0.));
#46386=DIRECTION('',(0.,1.,0.));
#46387=DIRECTION('',(6.19544098563145E-17,-1.,0.));
#46388=DIRECTION('',(1.,4.33680868994203E-15,0.));
#46389=DIRECTION('',(1.,0.,0.));
#46390=DIRECTION('',(1.,0.,0.));
#46391=DIRECTION('',(-1.,4.33680868994203E-15,0.));
#46392=DIRECTION('',(-6.19544098563145E-17,-1.,0.));
#46393=DIRECTION('',(-1.,4.33680868994203E-15,0.));
#46394=DIRECTION('',(-1.,6.08674903851511E-17,0.));
#46395=DIRECTION('',(-1.,6.08674903851511E-17,0.));
#46396=DIRECTION('',(1.,4.33680868994203E-15,0.));
#46397=DIRECTION('center_axis',(0.,1.,0.));
#46398=DIRECTION('ref_axis',(0.,0.,1.));
#46399=DIRECTION('',(0.,0.,-1.));
#46400=DIRECTION('',(1.,0.,0.));
#46401=DIRECTION('',(0.,0.,-1.));
#46402=DIRECTION('center_axis',(-1.,8.46206573647223E-17,0.));
#46403=DIRECTION('ref_axis',(-8.46206573647223E-17,-1.,0.));
#46404=DIRECTION('',(0.,0.,-1.));
#46405=DIRECTION('',(8.46206573647223E-17,1.,0.));
#46406=DIRECTION('center_axis',(-5.9818050895752E-17,1.,0.));
#46407=DIRECTION('ref_axis',(-1.,-5.9818050895752E-17,0.));
#46408=DIRECTION('',(0.,0.,-1.));
#46409=DIRECTION('',(1.,5.9818050895752E-17,0.));
#46410=DIRECTION('center_axis',(-1.,0.,0.));
#46411=DIRECTION('ref_axis',(0.,0.,1.));
#46412=DIRECTION('',(0.,1.,0.));
#46413=DIRECTION('center_axis',(0.,0.,1.));
#46414=DIRECTION('ref_axis',(1.,0.,0.));
#46415=DIRECTION('',(0.,1.,0.));
#46416=DIRECTION('',(1.,-6.42490176287706E-17,0.));
#46417=DIRECTION('',(0.,-1.,0.));
#46418=DIRECTION('',(-1.,0.,0.));
#46419=DIRECTION('center_axis',(6.08674903851511E-17,1.,0.));
#46420=DIRECTION('ref_axis',(-1.,6.08674903851511E-17,0.));
#46421=DIRECTION('center_axis',(-6.08674903851511E-17,-1.,0.));
#46422=DIRECTION('ref_axis',(-1.,6.08674903851511E-17,0.));
#46423=DIRECTION('center_axis',(-6.08674903851511E-17,-1.,0.));
#46424=DIRECTION('ref_axis',(-1.,6.08674903851511E-17,0.));
#46425=DIRECTION('',(2.31296463463574E-16,-1.40784352659886E-32,-1.));
#46426=DIRECTION('',(-0.0817503058163819,2.70504095639686E-16,0.99665284201618));
#46427=DIRECTION('',(0.427528579403957,-1.41465197685674E-15,0.904001832848161));
#46428=DIRECTION('',(-0.427528579403968,0.,-0.904001832848156));
#46429=DIRECTION('',(0.0817503058163822,0.,-0.99665284201618));
#46430=DIRECTION('',(0.,0.,1.));
#46431=DIRECTION('',(0.,0.,1.));
#46432=DIRECTION('',(-0.0817503058163822,0.,-0.99665284201618));
#46433=DIRECTION('',(0.427528579403968,0.,-0.904001832848156));
#46434=DIRECTION('',(-0.427528579403957,-1.41465197685674E-15,0.904001832848161));
#46435=DIRECTION('',(0.0817503058163819,2.70504095639686E-16,0.99665284201618));
#46436=DIRECTION('',(-2.31296463463574E-16,1.40784352659886E-32,1.));
#46437=DIRECTION('center_axis',(1.,0.,0.));
#46438=DIRECTION('ref_axis',(0.,0.,-1.));
#46439=DIRECTION('',(-6.19544098563145E-17,-1.,0.));
#46440=DIRECTION('',(0.,0.,1.));
#46441=DIRECTION('center_axis',(0.,-1.,0.));
#46442=DIRECTION('ref_axis',(0.,0.,-1.));
#46443=DIRECTION('center_axis',(0.,1.,0.));
#46444=DIRECTION('ref_axis',(0.,0.,-1.));
#46445=DIRECTION('center_axis',(0.,1.,0.));
#46446=DIRECTION('ref_axis',(0.,0.,-1.));
#46447=DIRECTION('',(2.31296463463574E-16,0.,-1.));
#46448=DIRECTION('',(0.0817503058163819,2.70504095639686E-16,0.99665284201618));
#46449=DIRECTION('',(-0.427528579403957,-1.41465197685674E-15,0.904001832848161));
#46450=DIRECTION('',(0.427528579403968,0.,-0.904001832848156));
#46451=DIRECTION('',(-0.0817503058163822,0.,-0.99665284201618));
#46452=DIRECTION('',(0.,0.,1.));
#46453=DIRECTION('',(0.0817503058163822,0.,-0.99665284201618));
#46454=DIRECTION('',(-0.427528579403968,0.,-0.904001832848156));
#46455=DIRECTION('',(0.427528579403957,-1.41465197685674E-15,0.904001832848161));
#46456=DIRECTION('',(-0.0817503058163819,2.70504095639686E-16,0.99665284201618));
#46457=DIRECTION('',(-2.31296463463574E-16,0.,1.));
#46458=DIRECTION('center_axis',(-1.,0.,0.));
#46459=DIRECTION('ref_axis',(0.,0.,1.));
#46460=DIRECTION('',(0.,-1.,0.));
#46461=DIRECTION('center_axis',(1.,0.,0.));
#46462=DIRECTION('ref_axis',(0.,0.,-1.));
#46463=DIRECTION('',(0.,1.,0.));
#46464=DIRECTION('center_axis',(0.,1.,0.));
#46465=DIRECTION('ref_axis',(0.,0.,1.));
#46466=DIRECTION('',(-1.,0.,0.));
#46467=DIRECTION('',(0.,0.,1.));
#46468=DIRECTION('center_axis',(0.,1.,0.));
#46469=DIRECTION('ref_axis',(0.,0.,1.));
#46470=DIRECTION('',(-1.,0.,0.));
#46471=DIRECTION('',(0.,0.,1.));
#46472=DIRECTION('center_axis',(0.,0.,1.));
#46473=DIRECTION('ref_axis',(1.,0.,0.));
#46474=DIRECTION('',(3.61400724161835E-16,1.,0.));
#46475=DIRECTION('',(1.,-3.61400724161835E-16,0.));
#46476=DIRECTION('',(4.33680868994202E-17,1.,0.));
#46477=DIRECTION('',(0.,1.,0.));
#46478=DIRECTION('',(4.33680868994202E-17,1.,0.));
#46479=DIRECTION('',(1.,-3.61400724161835E-16,0.));
#46480=DIRECTION('',(3.61400724161835E-16,1.,0.));
#46481=DIRECTION('center_axis',(1.,0.,0.));
#46482=DIRECTION('ref_axis',(0.,0.,-1.));
#46483=DIRECTION('center_axis',(1.,0.,0.));
#46484=DIRECTION('ref_axis',(0.,0.,-1.));
#46485=DIRECTION('',(0.,1.,0.));
#46486=DIRECTION('center_axis',(0.,1.,0.));
#46487=DIRECTION('ref_axis',(0.,0.,1.));
#46488=DIRECTION('',(-1.,0.,0.));
#46489=DIRECTION('',(0.,0.,1.));
#46490=DIRECTION('center_axis',(0.,1.,0.));
#46491=DIRECTION('ref_axis',(0.,0.,1.));
#46492=DIRECTION('',(-1.,0.,0.));
#46493=DIRECTION('',(0.,0.,1.));
#46494=DIRECTION('center_axis',(0.,0.,1.));
#46495=DIRECTION('ref_axis',(1.,0.,0.));
#46496=DIRECTION('',(3.46944695195361E-16,1.,0.));
#46497=DIRECTION('',(1.,-3.61400724161835E-16,0.));
#46498=DIRECTION('',(0.,1.,0.));
#46499=DIRECTION('',(0.,1.,0.));
#46500=DIRECTION('',(0.,1.,0.));
#46501=DIRECTION('',(1.,-3.61400724161835E-16,0.));
#46502=DIRECTION('',(3.46944695195361E-16,1.,0.));
#46503=DIRECTION('center_axis',(1.,0.,0.));
#46504=DIRECTION('ref_axis',(0.,0.,-1.));
#46505=DIRECTION('center_axis',(1.,-3.61400724161835E-16,0.));
#46506=DIRECTION('ref_axis',(3.61400724161835E-16,1.,0.));
#46507=DIRECTION('center_axis',(1.,-3.61400724161835E-16,0.));
#46508=DIRECTION('ref_axis',(-3.61400724161835E-16,-1.,0.));
#46509=DIRECTION('',(-1.61623317268703E-16,-0.44721359549996,0.894427190999915));
#46510=DIRECTION('',(3.61400724161835E-16,1.,0.));
#46511=DIRECTION('',(-1.61623317268703E-16,-0.447213595499958,-0.894427190999916));
#46512=DIRECTION('center_axis',(1.,-4.33680868994202E-17,0.));
#46513=DIRECTION('ref_axis',(4.33680868994202E-17,1.,0.));
#46514=DIRECTION('center_axis',(1.,-4.33680868994202E-17,0.));
#46515=DIRECTION('ref_axis',(4.33680868994202E-17,1.,0.));
#46516=DIRECTION('',(-1.93947980722443E-17,-0.447213595499958,-0.894427190999916));
#46517=DIRECTION('',(4.33680868994202E-17,1.,0.));
#46518=DIRECTION('',(-1.93947980722444E-17,-0.44721359549996,0.894427190999915));
#46519=DIRECTION('center_axis',(0.,0.,-1.));
#46520=DIRECTION('ref_axis',(-1.,0.,0.));
#46521=DIRECTION('',(-1.,0.,0.));
#46522=DIRECTION('',(-1.,0.,0.));
#46523=DIRECTION('center_axis',(1.,-3.46944695195361E-16,0.));
#46524=DIRECTION('ref_axis',(3.46944695195361E-16,1.,0.));
#46525=DIRECTION('center_axis',(1.,-3.46944695195361E-16,0.));
#46526=DIRECTION('ref_axis',(3.46944695195361E-16,1.,0.));
#46527=DIRECTION('',(-1.55158384577955E-16,-0.44721359549996,0.894427190999915));
#46528=DIRECTION('',(3.46944695195361E-16,1.,0.));
#46529=DIRECTION('',(-1.55158384577955E-16,-0.447213595499958,-0.894427190999916));
#46530=DIRECTION('center_axis',(1.,0.,0.));
#46531=DIRECTION('ref_axis',(0.,0.,-1.));
#46532=DIRECTION('center_axis',(1.,0.,0.));
#46533=DIRECTION('ref_axis',(0.,0.,-1.));
#46534=DIRECTION('',(0.,0.447213595499958,0.894427190999916));
#46535=DIRECTION('',(0.,1.,0.));
#46536=DIRECTION('',(0.,0.44721359549996,-0.894427190999915));
#46537=DIRECTION('center_axis',(0.,0.,-1.));
#46538=DIRECTION('ref_axis',(-1.,0.,0.));
#46539=DIRECTION('',(-1.,0.,0.));
#46540=DIRECTION('',(1.,0.,0.));
#46541=DIRECTION('center_axis',(0.,0.894427190999915,0.44721359549996));
#46542=DIRECTION('ref_axis',(0.,-0.44721359549996,0.894427190999915));
#46543=DIRECTION('center_axis',(0.,-0.894427190999916,0.447213595499958));
#46544=DIRECTION('ref_axis',(0.,-0.447213595499958,-0.894427190999916));
#46545=DIRECTION('center_axis',(0.,0.894427190999915,0.44721359549996));
#46546=DIRECTION('ref_axis',(0.,-0.44721359549996,0.894427190999915));
#46547=DIRECTION('center_axis',(0.,-0.894427190999916,0.447213595499958));
#46548=DIRECTION('ref_axis',(0.,-0.447213595499958,-0.894427190999916));
#46549=DIRECTION('center_axis',(1.,-3.61400724161835E-16,0.));
#46550=DIRECTION('ref_axis',(3.61400724161835E-16,1.,0.));
#46551=DIRECTION('center_axis',(1.,-3.61400724161835E-16,0.));
#46552=DIRECTION('ref_axis',(3.61400724161835E-16,1.,0.));
#46553=DIRECTION('center_axis',(-1.,6.19544098563145E-17,-2.31296463463574E-16));
#46554=DIRECTION('ref_axis',(-2.31296463463574E-16,0.,1.));
#46555=DIRECTION('',(-6.19544098563145E-17,-1.,0.));
#46556=DIRECTION('',(-6.19544098563145E-17,-1.,0.));
#46557=DIRECTION('center_axis',(1.,-6.19544098563145E-17,2.31296463463574E-16));
#46558=DIRECTION('ref_axis',(2.31296463463574E-16,0.,-1.));
#46559=DIRECTION('',(-6.19544098563145E-17,-1.,0.));
#46560=DIRECTION('',(-6.19544098563145E-17,-1.,0.));
#46561=DIRECTION('center_axis',(0.904001832848161,-5.60069000631345E-17,
-0.427528579403957));
#46562=DIRECTION('ref_axis',(-0.427528579403957,3.71975701883526E-34,-0.904001832848161));
#46563=DIRECTION('',(-6.19544098563145E-17,-1.,0.));
#46564=DIRECTION('center_axis',(0.99665284201618,-6.17470386587311E-17,
0.0817503058163819));
#46565=DIRECTION('ref_axis',(0.0817503058163819,8.42971361630042E-34,-0.99665284201618));
#46566=DIRECTION('center_axis',(-0.99665284201618,6.17470386587311E-17,
-0.0817503058163822));
#46567=DIRECTION('ref_axis',(-0.0817503058163822,-1.07140226946576E-35,
0.99665284201618));
#46568=DIRECTION('',(-6.19544098563145E-17,-1.,0.));
#46569=DIRECTION('center_axis',(-0.904001832848156,5.60069000631342E-17,
0.427528579403968));
#46570=DIRECTION('ref_axis',(0.427528579403968,-1.6530393860932E-34,0.904001832848156));
#46571=DIRECTION('center_axis',(-0.904001832848156,-5.60069000631342E-17,
-0.427528579403968));
#46572=DIRECTION('ref_axis',(-0.427528579403968,-1.6530393860932E-34,0.904001832848156));
#46573=DIRECTION('',(6.19544098563145E-17,-1.,0.));
#46574=DIRECTION('center_axis',(-0.99665284201618,-6.17470386587311E-17,
0.0817503058163822));
#46575=DIRECTION('ref_axis',(0.0817503058163822,-1.07140226946576E-35,0.99665284201618));
#46576=DIRECTION('center_axis',(0.99665284201618,6.17470386587311E-17,-0.0817503058163819));
#46577=DIRECTION('ref_axis',(-0.0817503058163819,8.42971361630042E-34,-0.99665284201618));
#46578=DIRECTION('',(6.19544098563145E-17,-1.,0.));
#46579=DIRECTION('center_axis',(0.904001832848161,5.60069000631345E-17,
0.427528579403957));
#46580=DIRECTION('ref_axis',(0.427528579403957,3.71975701883526E-34,-0.904001832848161));
#46581=DIRECTION('center_axis',(1.,0.,0.));
#46582=DIRECTION('ref_axis',(0.,0.,-1.));
#46583=DIRECTION('',(0.,0.,-1.));
#46584=DIRECTION('',(0.,0.,-1.));
#46585=DIRECTION('center_axis',(0.,1.,0.));
#46586=DIRECTION('ref_axis',(0.,0.,1.));
#46587=DIRECTION('',(0.,0.,-1.));
#46588=DIRECTION('center_axis',(-1.,0.,0.));
#46589=DIRECTION('ref_axis',(0.,0.,1.));
#46590=DIRECTION('',(0.,0.,-1.));
#46591=DIRECTION('center_axis',(0.,-1.,0.));
#46592=DIRECTION('ref_axis',(0.,0.,-1.));
#46593=DIRECTION('center_axis',(0.,1.,0.));
#46594=DIRECTION('ref_axis',(1.,0.,0.));
#46595=DIRECTION('center_axis',(0.,0.,1.));
#46596=DIRECTION('ref_axis',(-1.,0.,0.));
#46597=DIRECTION('center_axis',(0.,-1.,0.));
#46598=DIRECTION('ref_axis',(1.,0.,4.44089209850063E-16));
#46599=DIRECTION('center_axis',(5.55111512312578E-16,0.,-1.));
#46600=DIRECTION('ref_axis',(-1.,0.,-5.55111512312578E-16));
#57979=CARTESIAN_POINT('',(0.,0.,0.));
#57980=CARTESIAN_POINT('Origin',(-1.03877763349493,4.27252044680983E-8,
-2.34921160237358));
#57981=CARTESIAN_POINT('',(-7.78877763349493,4.6250000427252,-2.34921160237359));
#57982=CARTESIAN_POINT('',(-7.78877763349493,-4.6249999572748,-2.34921160237358));
#57983=CARTESIAN_POINT('',(-7.78877763349493,4.6250000427252,-2.34921160237358));
#57984=CARTESIAN_POINT('',(5.71122236650507,4.6250000427252,-2.34921160237359));
#57985=CARTESIAN_POINT('',(-7.78877763349493,4.6250000427252,-2.34921160237358));
#57986=CARTESIAN_POINT('',(5.71122236650507,-4.6249999572748,-2.34921160237359));
#57987=CARTESIAN_POINT('',(5.71122236650507,4.6250000427252,-2.34921160237358));
#57988=CARTESIAN_POINT('',(-7.78877763349493,-4.6249999572748,-2.34921160237358));
#57989=CARTESIAN_POINT('Origin',(-1.03877763349493,4.27252044680983E-8,
-5.84921160237358));
#57990=CARTESIAN_POINT('',(-7.78877763349493,-4.62499995727479,-5.84921160237358));
#57991=CARTESIAN_POINT('',(5.71122236650507,-4.6249999572748,-5.84921160237358));
#57992=CARTESIAN_POINT('',(-7.78877763349493,-4.62499995727479,-5.84921160237358));
#57993=CARTESIAN_POINT('',(5.71122236650507,4.6250000427252,-5.84921160237359));
#57994=CARTESIAN_POINT('',(5.71122236650507,-4.6249999572748,-5.84921160237358));
#57995=CARTESIAN_POINT('',(-7.78877763349493,4.6250000427252,-5.84921160237358));
#57996=CARTESIAN_POINT('',(-7.78877763349493,4.6250000427252,-5.84921160237358));
#57997=CARTESIAN_POINT('',(-7.78877763349493,-4.62499995727479,-5.84921160237358));
#57998=CARTESIAN_POINT('Origin',(-7.78877763349493,-4.62499995727479,-22.4641894514267));
#57999=CARTESIAN_POINT('',(5.71122236650507,-4.6249999572748,-22.4641894514267));
#58000=CARTESIAN_POINT('',(-7.78877763349493,-4.62499995727479,-22.4641894514267));
#58001=CARTESIAN_POINT('Origin',(-7.78877763349493,-4.62499995727479,-22.4641894514267));
#58002=CARTESIAN_POINT('',(-7.78877763349493,4.6250000427252,-22.4641894514267));
#58003=CARTESIAN_POINT('Origin',(-7.78877763349493,4.6250000427252,-22.4641894514267));
#58004=CARTESIAN_POINT('',(5.71122236650507,4.6250000427252,-22.4641894514267));
#58005=CARTESIAN_POINT('Origin',(5.71122236650507,-4.6249999572748,-22.4641894514267));
#58006=CARTESIAN_POINT('Origin',(-8.28877763349493,4.2725226612629E-8,-10.3492116023736));
#58007=CARTESIAN_POINT('',(-1.53877763349493,-0.999999957274778,-10.3492116023736));
#58008=CARTESIAN_POINT('Origin',(-1.53877763349493,4.27252241731742E-8,
-10.3492116023736));
#58009=CARTESIAN_POINT('',(-0.538777633494928,-0.999999957274778,-10.3492116023736));
#58010=CARTESIAN_POINT('',(-8.28877763349493,-0.999999957274775,-10.3492116023736));
#58011=CARTESIAN_POINT('Origin',(-0.538777633494929,4.27252238117734E-8,
-10.3492116023736));
#58012=CARTESIAN_POINT('Origin',(-8.28877763349493,4.2725226612629E-8,-10.3492116023736));
#58013=CARTESIAN_POINT('',(-6.53877763349493,-0.999999957274776,-10.3492116023736));
#58014=CARTESIAN_POINT('Origin',(-6.53877763349493,4.27252259801778E-8,
-10.3492116023736));
#58015=CARTESIAN_POINT('',(-5.53877763349493,-0.999999957274776,-10.3492116023736));
#58016=CARTESIAN_POINT('',(-8.28877763349493,-0.999999957274775,-10.3492116023736));
#58017=CARTESIAN_POINT('Origin',(-5.53877763349493,4.27252256187771E-8,
-10.3492116023736));
#58018=CARTESIAN_POINT('Origin',(12.9485298756357,4.6250000427252,55.4311528842592));
#58019=CARTESIAN_POINT('',(-7.78877763349493,4.6250000427252,3.41227095402391));
#58020=CARTESIAN_POINT('',(5.71122236650507,4.6250000427252,-0.0992116023735834));
#58021=CARTESIAN_POINT('Origin',(12.9485298756357,4.6250000427252,55.4311528842592));
#58022=CARTESIAN_POINT('',(-7.78877763349493,-4.6249999572748,3.41227095402391));
#58023=CARTESIAN_POINT('',(-7.78877763349493,4.6250000427252,3.41227095402391));
#58024=CARTESIAN_POINT('',(5.71122236650507,-4.6249999572748,-0.0992116023735834));
#58025=CARTESIAN_POINT('Origin',(12.9485298756357,-4.6249999572748,55.4311528842592));
#58026=CARTESIAN_POINT('',(5.71122236650507,4.6250000427252,-0.0992116023735834));
#58027=CARTESIAN_POINT('Origin',(-0.0387776334949297,-3.74999995727479,
-6.34921160237358));
#58028=CARTESIAN_POINT('',(-0.53877763349493,-3.74999995727479,-6.34921160237358));
#58029=CARTESIAN_POINT('',(-0.53877763349493,-3.74999995727479,-6.09921160237358));
#58030=CARTESIAN_POINT('',(-0.53877763349493,-3.74999995727479,-6.34921160237358));
#58031=CARTESIAN_POINT('',(-0.0387776334949297,-3.74999995727479,-6.34921160237358));
#58032=CARTESIAN_POINT('',(-0.0387776334949297,-3.74999995727479,-6.34921160237358));
#58033=CARTESIAN_POINT('',(-0.0387776334949297,-3.74999995727479,-6.09921160237358));
#58034=CARTESIAN_POINT('',(-0.0387776334949297,-3.74999995727479,-6.34921160237358));
#58035=CARTESIAN_POINT('',(-0.0387776334949297,-3.74999995727479,-6.09921160237358));
#58036=CARTESIAN_POINT('Origin',(-0.0387776334949297,3.75000004272521,-6.34921160237358));
#58037=CARTESIAN_POINT('',(-0.0387776334949297,3.75000004272521,-6.34921160237358));
#58038=CARTESIAN_POINT('',(-0.538777633494927,3.75000004272521,-6.34921160237358));
#58039=CARTESIAN_POINT('',(-0.0387776334949297,3.75000004272521,-6.34921160237358));
#58040=CARTESIAN_POINT('',(-0.53877763349493,3.75000004272521,-6.09921160237358));
#58041=CARTESIAN_POINT('',(-0.53877763349493,3.75000004272521,-6.34921160237358));
#58042=CARTESIAN_POINT('',(-0.0387776334949297,3.75000004272521,-6.09921160237358));
#58043=CARTESIAN_POINT('',(-0.0387776334949297,3.75000004272521,-6.09921160237358));
#58044=CARTESIAN_POINT('',(-0.0387776334949297,3.75000004272521,-6.34921160237358));
#58045=CARTESIAN_POINT('Origin',(-0.0387776334949297,-3.74999995727479,
-6.34921160237358));
#58046=CARTESIAN_POINT('',(-0.53877763349493,-3.74999995727479,-10.0992116023736));
#58047=CARTESIAN_POINT('',(-0.53877763349493,-3.74999995727479,-13.0992116023736));
#58048=CARTESIAN_POINT('',(-1.53877763349493,-3.74999995727479,-6.09921160237358));
#58049=CARTESIAN_POINT('',(-0.0387776334949297,-3.74999995727479,-6.09921160237358));
#58050=CARTESIAN_POINT('',(-1.53877763349493,-3.74999995727479,-6.34921160237358));
#58051=CARTESIAN_POINT('',(-1.53877763349493,-3.74999995727479,-6.34921160237358));
#58052=CARTESIAN_POINT('',(-1.53877763349493,-3.74999995727479,-10.0992116023736));
#58053=CARTESIAN_POINT('',(-1.53877763349493,-3.74999995727479,-13.0992116023736));
#58054=CARTESIAN_POINT('',(6.21122236650507,-3.74999995727479,-10.0992116023736));
#58055=CARTESIAN_POINT('Origin',(-0.0387776334949297,3.75000004272521,-6.34921160237358));
#58056=CARTESIAN_POINT('',(-0.538777633494927,3.75000004272521,-10.0992116023736));
#58057=CARTESIAN_POINT('',(-0.538777633494927,3.75000004272521,-13.0992116023736));
#58058=CARTESIAN_POINT('',(-1.53877763349493,3.75000004272521,-10.0992116023736));
#58059=CARTESIAN_POINT('',(6.21122236650507,3.75000004272521,-10.0992116023736));
#58060=CARTESIAN_POINT('',(-1.53877763349493,3.75000004272521,-6.34921160237358));
#58061=CARTESIAN_POINT('',(-1.53877763349493,3.75000004272521,-13.0992116023736));
#58062=CARTESIAN_POINT('',(-1.53877763349493,3.75000004272521,-6.09921160237358));
#58063=CARTESIAN_POINT('',(-1.53877763349493,3.75000004272521,-6.34921160237358));
#58064=CARTESIAN_POINT('',(-0.0387776334949297,3.75000004272521,-6.09921160237358));
#58065=CARTESIAN_POINT('Origin',(-5.03877763349493,3.75000004272521,-6.34921160237358));
#58066=CARTESIAN_POINT('',(-5.03877763349493,3.75000004272521,-6.34921160237358));
#58067=CARTESIAN_POINT('',(-5.53877763349493,3.75000004272521,-6.34921160237358));
#58068=CARTESIAN_POINT('',(-5.03877763349493,3.75000004272521,-6.34921160237358));
#58069=CARTESIAN_POINT('',(-5.53877763349493,3.75000004272521,-6.09921160237358));
#58070=CARTESIAN_POINT('',(-5.53877763349493,3.75000004272521,-6.34921160237358));
#58071=CARTESIAN_POINT('',(-5.03877763349493,3.75000004272521,-6.09921160237358));
#58072=CARTESIAN_POINT('',(-5.03877763349493,3.75000004272521,-6.09921160237358));
#58073=CARTESIAN_POINT('',(-5.03877763349493,3.75000004272521,-6.34921160237358));
#58074=CARTESIAN_POINT('Origin',(-5.03877763349493,-3.74999995727479,-6.34921160237358));
#58075=CARTESIAN_POINT('',(-5.53877763349493,-3.74999995727479,-6.34921160237358));
#58076=CARTESIAN_POINT('',(-5.53877763349493,-3.74999995727479,-6.09921160237358));
#58077=CARTESIAN_POINT('',(-5.53877763349493,-3.74999995727479,-6.34921160237358));
#58078=CARTESIAN_POINT('',(-5.03877763349493,-3.74999995727479,-6.34921160237358));
#58079=CARTESIAN_POINT('',(-5.03877763349493,-3.74999995727479,-6.34921160237358));
#58080=CARTESIAN_POINT('',(-5.03877763349493,-3.74999995727479,-6.09921160237358));
#58081=CARTESIAN_POINT('',(-5.03877763349493,-3.74999995727479,-6.34921160237358));
#58082=CARTESIAN_POINT('',(-5.03877763349493,-3.74999995727479,-6.09921160237358));
#58083=CARTESIAN_POINT('Origin',(-5.03877763349493,3.75000004272521,-6.34921160237358));
#58084=CARTESIAN_POINT('',(-5.53877763349493,3.75000004272521,-10.0992116023736));
#58085=CARTESIAN_POINT('',(-5.53877763349493,3.75000004272521,-13.0992116023736));
#58086=CARTESIAN_POINT('',(-6.53877763349493,3.75000004272521,-10.0992116023736));
#58087=CARTESIAN_POINT('',(6.21122236650507,3.75000004272521,-10.0992116023736));
#58088=CARTESIAN_POINT('',(-6.53877763349493,3.75000004272521,-6.34921160237358));
#58089=CARTESIAN_POINT('',(-6.53877763349493,3.75000004272521,-13.0992116023736));
#58090=CARTESIAN_POINT('',(-6.53877763349493,3.75000004272521,-6.09921160237358));
#58091=CARTESIAN_POINT('',(-6.53877763349493,3.75000004272521,-6.34921160237358));
#58092=CARTESIAN_POINT('',(-5.03877763349493,3.75000004272521,-6.09921160237358));
#58093=CARTESIAN_POINT('Origin',(-5.03877763349493,-3.74999995727479,-6.34921160237358));
#58094=CARTESIAN_POINT('',(-5.53877763349493,-3.74999995727479,-10.0992116023736));
#58095=CARTESIAN_POINT('',(-5.53877763349493,-3.74999995727479,-13.0992116023736));
#58096=CARTESIAN_POINT('',(-6.53877763349493,-3.74999995727479,-6.09921160237358));
#58097=CARTESIAN_POINT('',(-5.03877763349493,-3.74999995727479,-6.09921160237358));
#58098=CARTESIAN_POINT('',(-6.53877763349493,-3.74999995727479,-6.34921160237358));
#58099=CARTESIAN_POINT('',(-6.53877763349493,-3.74999995727479,-6.34921160237358));
#58100=CARTESIAN_POINT('',(-6.53877763349493,-3.74999995727479,-10.0992116023736));
#58101=CARTESIAN_POINT('',(-6.53877763349493,-3.74999995727479,-13.0992116023736));
#58102=CARTESIAN_POINT('',(6.21122236650507,-3.74999995727479,-10.0992116023736));
#58103=CARTESIAN_POINT('Origin',(-1.03877763349493,4.27252044680983E-8,
-6.09921160237358));
#58104=CARTESIAN_POINT('',(6.08622236650508,-4.9999999572748,-6.09921160237358));
#58105=CARTESIAN_POINT('',(-8.16377763349493,-4.99999995727479,-6.09921160237358));
#58106=CARTESIAN_POINT('',(6.08622236650508,-4.9999999572748,-6.09921160237358));
#58107=CARTESIAN_POINT('',(-8.16377763349493,5.00000004272521,-6.09921160237358));
#58108=CARTESIAN_POINT('',(-8.16377763349493,-4.99999995727479,-6.09921160237358));
#58109=CARTESIAN_POINT('',(6.08622236650508,5.00000004272521,-6.09921160237358));
#58110=CARTESIAN_POINT('',(-8.16377763349493,5.00000004272521,-6.09921160237358));
#58111=CARTESIAN_POINT('',(6.08622236650508,5.00000004272521,-6.09921160237358));
#58112=CARTESIAN_POINT('',(-2.03877763349493,-3.74999995727479,-6.09921160237358));
#58113=CARTESIAN_POINT('',(-2.03877763349493,3.75000004272521,-6.09921160237358));
#58114=CARTESIAN_POINT('',(-2.03877763349493,-3.74999995727479,-6.09921160237358));
#58115=CARTESIAN_POINT('',(-0.0387776334949297,-3.74999995727479,-6.09921160237358));
#58116=CARTESIAN_POINT('',(-0.0387776334949297,-3.74999995727479,-6.09921160237358));
#58117=CARTESIAN_POINT('',(-0.0387776334949297,3.75000004272521,-6.09921160237358));
#58118=CARTESIAN_POINT('',(-7.03877763349493,-3.74999995727479,-6.09921160237358));
#58119=CARTESIAN_POINT('',(-7.03877763349493,3.75000004272521,-6.09921160237358));
#58120=CARTESIAN_POINT('',(-7.03877763349493,-3.74999995727479,-6.09921160237358));
#58121=CARTESIAN_POINT('',(-5.03877763349493,-3.74999995727479,-6.09921160237358));
#58122=CARTESIAN_POINT('',(-5.03877763349493,-3.74999995727479,-6.09921160237358));
#58123=CARTESIAN_POINT('',(-5.03877763349493,3.75000004272521,-6.09921160237358));
#58124=CARTESIAN_POINT('Origin',(-1.03877763349493,4.27252044680983E-8,
-1.09921160237358));
#58125=CARTESIAN_POINT('',(-8.28877763349493,5.1250000427252,-1.09921160237358));
#58126=CARTESIAN_POINT('',(6.21122236650508,5.12500004272521,-1.09921160237358));
#58127=CARTESIAN_POINT('',(-8.28877763349493,5.1250000427252,-1.09921160237358));
#58128=CARTESIAN_POINT('',(6.21122236650507,-5.1249999572748,-1.09921160237358));
#58129=CARTESIAN_POINT('',(6.21122236650507,-5.1249999572748,-1.09921160237358));
#58130=CARTESIAN_POINT('',(-8.28877763349493,-5.1249999572748,-1.09921160237358));
#58131=CARTESIAN_POINT('',(-8.28877763349493,-5.1249999572748,-1.09921160237358));
#58132=CARTESIAN_POINT('',(-8.28877763349493,-5.1249999572748,-1.09921160237358));
#58133=CARTESIAN_POINT('',(6.08622236650507,5.00000004272521,-1.09921160237358));
#58134=CARTESIAN_POINT('',(6.08622236650507,-4.99999995727479,-1.09921160237358));
#58135=CARTESIAN_POINT('',(6.08622236650507,5.00000004272521,-1.09921160237358));
#58136=CARTESIAN_POINT('',(5.88622236650507,5.00000004272521,-1.09921160237358));
#58137=CARTESIAN_POINT('',(6.08622236650507,5.00000004272521,-1.09921160237358));
#58138=CARTESIAN_POINT('',(-1.03877763349493,5.00000004272521,-1.09921160237358));
#58139=CARTESIAN_POINT('',(-8.16377763349493,5.00000004272521,-1.09921160237358));
#58140=CARTESIAN_POINT('',(-7.96377763349493,5.00000004272521,-1.09921160237358));
#58141=CARTESIAN_POINT('',(-8.16377763349493,5.00000004272521,-1.09921160237358));
#58142=CARTESIAN_POINT('',(-8.16377763349493,5.00000004272521,-1.09921160237358));
#58143=CARTESIAN_POINT('',(-8.16377763349493,5.00000004272521,-1.09921160237358));
#58144=CARTESIAN_POINT('',(-8.16377763349493,-4.99999995727479,-1.09921160237358));
#58145=CARTESIAN_POINT('',(-8.16377763349493,5.00000004272521,-1.09921160237358));
#58146=CARTESIAN_POINT('',(-7.96377763349493,-4.99999995727479,-1.09921160237358));
#58147=CARTESIAN_POINT('',(-8.16377763349493,-4.99999995727479,-1.09921160237358));
#58148=CARTESIAN_POINT('',(-1.03877763349493,-4.99999995727479,-1.09921160237358));
#58149=CARTESIAN_POINT('',(6.08622236650508,-4.9999999572748,-1.09921160237358));
#58150=CARTESIAN_POINT('',(5.88622236650507,-4.99999995727479,-1.09921160237358));
#58151=CARTESIAN_POINT('',(6.08622236650508,-4.9999999572748,-1.09921160237358));
#58152=CARTESIAN_POINT('',(6.08622236650507,-4.99999995727479,-1.09921160237358));
#58153=CARTESIAN_POINT('Origin',(-8.28877763349493,-5.1249999572748,-0.349211602373583));
#58154=CARTESIAN_POINT('',(6.21122236650507,-5.1249999572748,-0.349211602373583));
#58155=CARTESIAN_POINT('',(6.21122236650507,-5.1249999572748,-0.349211602373583));
#58156=CARTESIAN_POINT('',(-8.28877763349493,-5.1249999572748,-0.349211602373583));
#58157=CARTESIAN_POINT('',(-8.28877763349493,-5.1249999572748,-0.349211602373583));
#58158=CARTESIAN_POINT('',(-8.28877763349493,-5.1249999572748,-0.349211602373583));
#58159=CARTESIAN_POINT('Origin',(6.21122236650507,-5.1249999572748,-0.349211602373583));
#58160=CARTESIAN_POINT('',(6.21122236650508,5.12500004272521,-0.349211602373583));
#58161=CARTESIAN_POINT('',(6.21122236650508,5.12500004272521,-0.349211602373583));
#58162=CARTESIAN_POINT('',(6.21122236650507,-5.1249999572748,-0.349211602373583));
#58163=CARTESIAN_POINT('Origin',(-8.28877763349493,5.1250000427252,-0.349211602373583));
#58164=CARTESIAN_POINT('',(-8.28877763349493,5.1250000427252,-0.349211602373583));
#58165=CARTESIAN_POINT('',(-8.28877763349493,5.1250000427252,-0.349211602373583));
#58166=CARTESIAN_POINT('',(-8.28877763349493,5.1250000427252,-0.349211602373583));
#58167=CARTESIAN_POINT('Origin',(-8.28877763349493,-5.1249999572748,-0.349211602373583));
#58168=CARTESIAN_POINT('',(-8.28877763349493,-5.1249999572748,-0.349211602373583));
#58169=CARTESIAN_POINT('Origin',(-1.03877763349493,4.27252044680983E-8,
-0.349211602373583));
#58170=CARTESIAN_POINT('',(5.71122236650507,-4.6249999572748,-0.349211602373583));
#58171=CARTESIAN_POINT('',(5.71122236650507,4.6250000427252,-0.349211602373583));
#58172=CARTESIAN_POINT('',(5.71122236650507,-4.6249999572748,-0.349211602373583));
#58173=CARTESIAN_POINT('',(-7.78877763349493,-4.62499995727479,-0.349211602373583));
#58174=CARTESIAN_POINT('',(-7.78877763349493,-4.62499995727479,-0.349211602373583));
#58175=CARTESIAN_POINT('',(-7.78877763349493,4.6250000427252,-0.349211602373583));
#58176=CARTESIAN_POINT('',(-7.78877763349493,-4.62499995727479,-0.349211602373583));
#58177=CARTESIAN_POINT('',(-7.78877763349493,4.6250000427252,-0.349211602373583));
#58178=CARTESIAN_POINT('Origin',(6.08622236650508,-4.9999999572748,-6.09921160237358));
#58179=CARTESIAN_POINT('',(-1.53877763349493,-4.99999995727479,-1.59921160237358));
#58180=CARTESIAN_POINT('Origin',(-1.03877763349493,-4.99999995727479,-1.59921160237358));
#58181=CARTESIAN_POINT('Origin',(-1.03877763349493,-4.99999995727479,-1.59921160237358));
#58182=CARTESIAN_POINT('',(-7.96377763349493,-4.99999995727479,-4.84921160237358));
#58183=CARTESIAN_POINT('',(-7.96377763349493,-4.99999995727479,-6.09921160237359));
#58184=CARTESIAN_POINT('',(-8.2259070743313,-4.99999995727479,-1.65347979957788));
#58185=CARTESIAN_POINT('',(-8.2259070743313,-4.99999995727479,-1.65347979957788));
#58186=CARTESIAN_POINT('',(-7.96377763349493,-4.99999995727479,-1.09921160237358));
#58187=CARTESIAN_POINT('',(-8.4259070743313,-4.99999995727479,-1.65347979957787));
#58188=CARTESIAN_POINT('',(-8.4259070743313,-4.99999995727479,-1.65347979957787));
#58189=CARTESIAN_POINT('',(-8.16377763349493,-4.99999995727479,-4.84921160237358));
#58190=CARTESIAN_POINT('',(-8.16377763349493,-4.99999995727479,-4.84921160237358));
#58191=CARTESIAN_POINT('',(-8.16377763349493,-4.99999995727479,-6.09921160237358));
#58192=CARTESIAN_POINT('',(6.08622236650507,-4.99999995727479,-4.84921160237358));
#58193=CARTESIAN_POINT('',(6.08622236650508,-4.9999999572748,-6.09921160237358));
#58194=CARTESIAN_POINT('',(6.34835180734145,-4.99999995727479,-1.65347979957787));
#58195=CARTESIAN_POINT('',(6.08622236650507,-4.99999995727479,-4.84921160237358));
#58196=CARTESIAN_POINT('',(6.34835180734145,-4.99999995727479,-1.65347979957787));
#58197=CARTESIAN_POINT('',(6.14835180734145,-4.99999995727479,-1.65347979957788));
#58198=CARTESIAN_POINT('',(5.88622236650507,-4.99999995727479,-1.09921160237358));
#58199=CARTESIAN_POINT('',(5.88622236650507,-4.99999995727479,-4.84921160237358));
#58200=CARTESIAN_POINT('',(6.14835180734145,-4.99999995727479,-1.65347979957788));
#58201=CARTESIAN_POINT('',(5.88622236650507,-4.9999999572748,-6.09921160237358));
#58202=CARTESIAN_POINT('Origin',(-8.16377763349493,-4.99999995727479,-6.09921160237358));
#58203=CARTESIAN_POINT('',(-8.16377763349493,5.00000004272521,-4.84921160237358));
#58204=CARTESIAN_POINT('',(-8.16377763349493,5.12500004272521,-4.84921160237358));
#58205=CARTESIAN_POINT('',(-8.16377763349493,5.00000004272521,-6.09921160237358));
#58206=CARTESIAN_POINT('Origin',(-8.16377763349493,5.00000004272521,-6.09921160237358));
#58207=CARTESIAN_POINT('',(-1.53877763349493,5.00000004272521,-1.59921160237358));
#58208=CARTESIAN_POINT('Origin',(-1.03877763349493,5.00000004272521,-1.59921160237358));
#58209=CARTESIAN_POINT('Origin',(-1.03877763349493,5.00000004272521,-1.59921160237358));
#58210=CARTESIAN_POINT('',(5.88622236650507,5.00000004272521,-4.84921160237358));
#58211=CARTESIAN_POINT('',(5.88622236650507,5.00000004272521,-6.09921160237358));
#58212=CARTESIAN_POINT('',(6.14835180734144,5.00000004272521,-1.65347979957788));
#58213=CARTESIAN_POINT('',(6.14835180734144,5.00000004272521,-1.65347979957788));
#58214=CARTESIAN_POINT('',(5.88622236650507,5.00000004272521,-1.09921160237358));
#58215=CARTESIAN_POINT('',(6.34835180734145,5.00000004272521,-1.65347979957787));
#58216=CARTESIAN_POINT('',(6.34835180734145,5.00000004272521,-1.65347979957787));
#58217=CARTESIAN_POINT('',(6.08622236650507,5.00000004272521,-4.84921160237358));
#58218=CARTESIAN_POINT('',(6.08622236650507,5.00000004272521,-4.84921160237358));
#58219=CARTESIAN_POINT('',(6.08622236650508,5.00000004272521,-6.09921160237358));
#58220=CARTESIAN_POINT('',(-8.4259070743313,5.00000004272521,-1.65347979957787));
#58221=CARTESIAN_POINT('',(-8.16377763349493,5.00000004272521,-4.84921160237358));
#58222=CARTESIAN_POINT('',(-8.4259070743313,5.00000004272521,-1.65347979957787));
#58223=CARTESIAN_POINT('',(-8.2259070743313,5.00000004272521,-1.65347979957788));
#58224=CARTESIAN_POINT('',(-7.96377763349493,5.00000004272521,-1.09921160237358));
#58225=CARTESIAN_POINT('',(-7.96377763349493,5.00000004272521,-4.84921160237358));
#58226=CARTESIAN_POINT('',(-8.2259070743313,5.00000004272521,-1.65347979957788));
#58227=CARTESIAN_POINT('',(-7.96377763349493,5.00000004272521,-6.09921160237358));
#58228=CARTESIAN_POINT('Origin',(6.08622236650508,5.00000004272521,-6.09921160237358));
#58229=CARTESIAN_POINT('',(6.08622236650508,5.00000004272521,-4.84921160237358));
#58230=CARTESIAN_POINT('Origin',(-0.0387776334949297,-3.74999995727479,
-6.34921160237358));
#58231=CARTESIAN_POINT('',(-0.0387776334949297,-3.74999995727479,-6.34921160237358));
#58232=CARTESIAN_POINT('Origin',(-0.0387776334949297,-3.74999995727479,
-6.34921160237358));
#58233=CARTESIAN_POINT('',(-2.03877763349493,-3.74999995727479,-6.34921160237358));
#58234=CARTESIAN_POINT('',(-1.53877763349493,-3.74999995727479,-6.34921160237358));
#58235=CARTESIAN_POINT('',(-2.03877763349493,-3.74999995727479,-6.34921160237358));
#58236=CARTESIAN_POINT('Origin',(-0.0387776334949297,3.75000004272521,-6.34921160237358));
#58237=CARTESIAN_POINT('',(-2.03877763349493,3.75000004272521,-6.34921160237358));
#58238=CARTESIAN_POINT('',(-1.53877763349493,3.75000004272521,-6.34921160237358));
#58239=CARTESIAN_POINT('',(-2.03877763349493,3.75000004272521,-6.34921160237358));
#58240=CARTESIAN_POINT('Origin',(-1.03877763349493,4.27252044680983E-8,
-6.34921160237358));
#58241=CARTESIAN_POINT('',(-0.538777633494929,-0.999999957274796,-6.34921160237358));
#58242=CARTESIAN_POINT('',(-0.53877763349493,-3.74999995727479,-6.34921160237358));
#58243=CARTESIAN_POINT('',(-1.53877763349493,-0.999999957274796,-6.34921160237358));
#58244=CARTESIAN_POINT('',(-8.28877763349493,-0.999999957274793,-6.34921160237358));
#58245=CARTESIAN_POINT('',(-1.53877763349493,-3.74999995727479,-6.34921160237358));
#58246=CARTESIAN_POINT('',(-2.03877763349493,-3.74999995727479,-6.34921160237358));
#58247=CARTESIAN_POINT('',(-1.53877763349493,1.0000000427252,-6.34921160237358));
#58248=CARTESIAN_POINT('',(-1.53877763349493,-3.74999995727479,-6.34921160237358));
#58249=CARTESIAN_POINT('',(-0.538777633494928,1.00000004272521,-6.34921160237358));
#58250=CARTESIAN_POINT('',(-8.28877763349493,1.00000004272521,-6.34921160237358));
#58251=CARTESIAN_POINT('',(-0.53877763349493,-3.74999995727479,-6.34921160237358));
#58252=CARTESIAN_POINT('Origin',(-2.03877763349493,-3.74999995727479,-6.34921160237358));
#58253=CARTESIAN_POINT('Origin',(-5.03877763349493,-3.74999995727479,-6.34921160237358));
#58254=CARTESIAN_POINT('',(-5.03877763349493,-3.74999995727479,-6.34921160237358));
#58255=CARTESIAN_POINT('Origin',(-5.03877763349493,-3.74999995727479,-6.34921160237358));
#58256=CARTESIAN_POINT('',(-7.03877763349493,-3.74999995727479,-6.34921160237358));
#58257=CARTESIAN_POINT('',(-6.53877763349493,-3.74999995727479,-6.34921160237358));
#58258=CARTESIAN_POINT('',(-7.03877763349493,-3.74999995727479,-6.34921160237358));
#58259=CARTESIAN_POINT('Origin',(-5.03877763349493,3.75000004272521,-6.34921160237358));
#58260=CARTESIAN_POINT('',(-7.03877763349493,3.75000004272521,-6.34921160237358));
#58261=CARTESIAN_POINT('',(-6.53877763349493,3.75000004272521,-6.34921160237358));
#58262=CARTESIAN_POINT('',(-7.03877763349493,3.75000004272521,-6.34921160237358));
#58263=CARTESIAN_POINT('Origin',(-1.03877763349493,4.27252044680983E-8,
-6.34921160237358));
#58264=CARTESIAN_POINT('',(-5.53877763349493,-0.999999957274794,-6.34921160237358));
#58265=CARTESIAN_POINT('',(-5.53877763349493,-3.74999995727479,-6.34921160237358));
#58266=CARTESIAN_POINT('',(-6.53877763349493,-0.999999957274796,-6.34921160237358));
#58267=CARTESIAN_POINT('',(-8.28877763349493,-0.999999957274793,-6.34921160237358));
#58268=CARTESIAN_POINT('',(-6.53877763349493,-3.74999995727479,-6.34921160237358));
#58269=CARTESIAN_POINT('',(-7.03877763349493,-3.74999995727479,-6.34921160237358));
#58270=CARTESIAN_POINT('',(-6.53877763349493,1.00000004272521,-6.34921160237358));
#58271=CARTESIAN_POINT('',(-6.53877763349493,-3.74999995727479,-6.34921160237358));
#58272=CARTESIAN_POINT('',(-5.53877763349493,1.00000004272521,-6.34921160237358));
#58273=CARTESIAN_POINT('',(-8.28877763349493,1.00000004272521,-6.34921160237358));
#58274=CARTESIAN_POINT('',(-5.53877763349493,-3.74999995727479,-6.34921160237358));
#58275=CARTESIAN_POINT('Origin',(-7.03877763349493,-3.74999995727479,-6.34921160237358));
#58276=CARTESIAN_POINT('Origin',(-0.538777633494929,4.2725204287398E-8,
-13.0992116023736));
#58277=CARTESIAN_POINT('Origin',(-0.538777633494929,4.27252151294197E-8,
-6.34921160237358));
#58278=CARTESIAN_POINT('',(-0.538777633494927,-2.24999995727479,-13.0992116023736));
#58279=CARTESIAN_POINT('',(-0.538777633494929,-1.79999995727478,-13.9992116023736));
#58280=CARTESIAN_POINT('',(-0.538777633494928,2.25000004272521,-13.0992116023736));
#58281=CARTESIAN_POINT('',(-0.538777633494929,4.2725204287398E-8,-13.0992116023736));
#58282=CARTESIAN_POINT('',(-0.538777633494928,1.80000004272521,-13.9992116023736));
#58283=CARTESIAN_POINT('Origin',(-1.53877763349493,4.27252044897824E-8,
-13.0992116023736));
#58284=CARTESIAN_POINT('Origin',(-1.53877763349493,4.27252154908204E-8,
-6.34921160237358));
#58285=CARTESIAN_POINT('',(-1.53877763349493,2.25000004272521,-13.0992116023736));
#58286=CARTESIAN_POINT('',(-1.53877763349493,1.80000004272521,-13.9992116023736));
#58287=CARTESIAN_POINT('',(-1.53877763349493,-2.24999995727479,-13.0992116023736));
#58288=CARTESIAN_POINT('',(-1.53877763349493,4.27252044897824E-8,-13.0992116023736));
#58289=CARTESIAN_POINT('',(-1.53877763349493,-1.79999995727478,-13.9992116023736));
#58290=CARTESIAN_POINT('Origin',(-1.03877763349493,4.27252044680983E-8,
-13.0992116023736));
#58291=CARTESIAN_POINT('',(6.21122236650507,2.25000004272521,-13.0992116023736));
#58292=CARTESIAN_POINT('',(6.21122236650507,-2.24999995727479,-13.0992116023736));
#58293=CARTESIAN_POINT('Origin',(-5.53877763349493,4.27252060293495E-8,
-13.0992116023736));
#58294=CARTESIAN_POINT('Origin',(-5.53877763349493,4.27252169364233E-8,
-6.34921160237358));
#58295=CARTESIAN_POINT('',(-5.53877763349493,-2.24999995727479,-13.0992116023736));
#58296=CARTESIAN_POINT('',(-5.53877763349493,-1.79999995727478,-13.9992116023736));
#58297=CARTESIAN_POINT('',(-5.53877763349493,2.25000004272521,-13.0992116023736));
#58298=CARTESIAN_POINT('',(-5.53877763349493,4.27252060293495E-8,-13.0992116023736));
#58299=CARTESIAN_POINT('',(-5.53877763349493,1.80000004272521,-13.9992116023736));
#58300=CARTESIAN_POINT('Origin',(-6.53877763349493,4.27252044680983E-8,
-13.0992116023736));
#58301=CARTESIAN_POINT('Origin',(-6.53877763349493,4.2725217297824E-8,-6.34921160237358));
#58302=CARTESIAN_POINT('',(-6.53877763349493,2.25000004272521,-13.0992116023736));
#58303=CARTESIAN_POINT('',(-6.53877763349493,3.75000004272521,-10.0992116023736));
#58304=CARTESIAN_POINT('',(-6.53877763349493,-2.24999995727479,-13.0992116023736));
#58305=CARTESIAN_POINT('',(-6.53877763349493,4.27252044680983E-8,-13.0992116023736));
#58306=CARTESIAN_POINT('',(-6.53877763349493,-3.74999995727479,-10.0992116023736));
#58307=CARTESIAN_POINT('Origin',(-1.03877763349493,4.27252044680983E-8,
-13.0992116023736));
#58308=CARTESIAN_POINT('',(-1.03877763349493,2.25000004272521,-13.0992116023736));
#58309=CARTESIAN_POINT('',(-1.03877763349493,-2.24999995727479,-13.0992116023736));
#58310=CARTESIAN_POINT('Origin',(6.21122236650507,-3.74999995727479,-10.0992116023736));
#58311=CARTESIAN_POINT('Origin',(6.21122236650507,3.75000004272521,-10.0992116023736));
#58312=CARTESIAN_POINT('Origin',(6.21122236650507,-3.74999995727479,-10.0992116023736));
#58313=CARTESIAN_POINT('Origin',(6.21122236650507,3.75000004272521,-10.0992116023736));
#58314=CARTESIAN_POINT('Origin',(-8.28877763349493,4.27252179302753E-8,
-6.34921160237358));
#58315=CARTESIAN_POINT('Origin',(-8.28877763349493,4.27252179302753E-8,
-6.34921160237358));
#58316=CARTESIAN_POINT('Origin',(5.88622236650507,5.12500004272521,-4.84921160237358));
#58317=CARTESIAN_POINT('',(5.88622236650507,5.12500004272521,-4.84921160237358));
#58318=CARTESIAN_POINT('',(5.88622236650507,5.12500004272521,-1.09921160237358));
#58319=CARTESIAN_POINT('Origin',(-7.96377763349493,5.12500004272521,-4.84921160237358));
#58320=CARTESIAN_POINT('',(-7.96377763349493,5.12500004272521,-1.09921160237358));
#58321=CARTESIAN_POINT('',(-7.96377763349493,5.12500004272521,-4.84921160237358));
#58322=CARTESIAN_POINT('Origin',(-7.96377763349493,5.00000004272521,-1.09921160237358));
#58323=CARTESIAN_POINT('',(-8.2259070743313,5.00000004272521,-1.65347979957788));
#58324=CARTESIAN_POINT('Origin',(-8.2259070743313,5.00000004272521,-1.65347979957788));
#58325=CARTESIAN_POINT('Origin',(-8.16377763349493,5.00000004272521,-4.84921160237358));
#58326=CARTESIAN_POINT('',(-8.4259070743313,5.00000004272521,-1.65347979957787));
#58327=CARTESIAN_POINT('Origin',(-8.4259070743313,5.00000004272521,-1.65347979957787));
#58328=CARTESIAN_POINT('Origin',(6.34835180734145,5.00000004272521,-1.65347979957787));
#58329=CARTESIAN_POINT('',(6.34835180734145,5.00000004272521,-1.65347979957787));
#58330=CARTESIAN_POINT('Origin',(6.08622236650507,5.00000004272521,-4.84921160237358));
#58331=CARTESIAN_POINT('Origin',(6.14835180734144,5.00000004272521,-1.65347979957788));
#58332=CARTESIAN_POINT('',(6.14835180734144,5.00000004272521,-1.65347979957788));
#58333=CARTESIAN_POINT('Origin',(5.88622236650507,5.00000004272521,-1.09921160237358));
#58334=CARTESIAN_POINT('Origin',(-7.78877763349493,4.6250000427252,-0.0992116023735834));
#58335=CARTESIAN_POINT('',(-7.78877763349493,-4.6249999572748,-0.0992116023735834));
#58336=CARTESIAN_POINT('',(-7.78877763349493,4.6250000427252,-0.0992116023735834));
#58337=CARTESIAN_POINT('Origin',(-7.78877763349493,-4.6249999572748,-0.0992116023735834));
#58338=CARTESIAN_POINT('',(5.71122236650507,-4.6249999572748,-0.0992116023735834));
#58339=CARTESIAN_POINT('Origin',(5.71122236650507,4.6250000427252,-0.0992116023735834));
#58340=CARTESIAN_POINT('',(5.71122236650507,4.6250000427252,-0.0992116023735834));
#58341=CARTESIAN_POINT('Origin',(-7.78877763349493,4.6250000427252,-0.0992116023735834));
#58342=CARTESIAN_POINT('Origin',(-1.03877763349493,-4.99999995727479,-1.59921160237358));
#58343=CARTESIAN_POINT('',(-1.03877763349493,-5.4999999572748,-1.59921160237358));
#58344=CARTESIAN_POINT('Origin',(-1.03877763349493,-4.99999995727479,-1.59921160237358));
#58345=CARTESIAN_POINT('Origin',(-1.03877763349493,5.00000004272521,-1.59921160237358));
#58346=CARTESIAN_POINT('',(-1.03877763349493,5.50000004272521,-1.59921160237358));
#58347=CARTESIAN_POINT('Origin',(-1.03877763349493,5.00000004272521,-1.59921160237358));
#65296=UNCERTAINTY_MEASURE_WITH_UNIT(LENGTH_MEASURE(0.01),#65305,
'DISTANCE_ACCURACY_VALUE',
'Maximum model space distance between geometric entities at asserted c
onnectivities');
#65298=UNCERTAINTY_MEASURE_WITH_UNIT(LENGTH_MEASURE(0.01),#65305,
'DISTANCE_ACCURACY_VALUE',
'Maximum model space distance between geometric entities at asserted c
onnectivities');
#65302=(
GEOMETRIC_REPRESENTATION_CONTEXT(3)
GLOBAL_UNCERTAINTY_ASSIGNED_CONTEXT((#65296))
GLOBAL_UNIT_ASSIGNED_CONTEXT((#65305,#65307,#65308))
REPRESENTATION_CONTEXT('','3D')
);
#65304=(
GEOMETRIC_REPRESENTATION_CONTEXT(3)
GLOBAL_UNCERTAINTY_ASSIGNED_CONTEXT((#65298))
GLOBAL_UNIT_ASSIGNED_CONTEXT((#65305,#65307,#65308))
REPRESENTATION_CONTEXT('','3D')
);
#65305=(
LENGTH_UNIT()
NAMED_UNIT(*)
SI_UNIT(.MILLI.,.METRE.)
);
#65307=(
NAMED_UNIT(*)
PLANE_ANGLE_UNIT()
SI_UNIT($,.RADIAN.)
);
#65308=(
NAMED_UNIT(*)
SI_UNIT($,.STERADIAN.)
SOLID_ANGLE_UNIT()
);
#65312=SHAPE_DEFINITION_REPRESENTATION(#65317,#65326);
#65317=PRODUCT_DEFINITION_SHAPE('',$,#65332);
#65326=SHAPE_REPRESENTATION('',(#41224),#65302);
#65328=PRODUCT_DEFINITION_CONTEXT('part definition',#65345,'design');
#65332=PRODUCT_DEFINITION('Swich_Predeterminado','Swich_Predeterminado',
#65337,#65328);
#65337=PRODUCT_DEFINITION_FORMATION('',$,#65350);
#65345=APPLICATION_CONTEXT(
'Core Data for Automotive Mechanical Design Process');
#65346=PRODUCT_CONTEXT('part definition',#65345,'mechanical');
#65350=PRODUCT('Swich_Predeterminado','Swich_Predeterminado',$,(#65346));
#65355=PRESENTATION_STYLE_ASSIGNMENT((#65360));
#65360=SURFACE_STYLE_USAGE(.BOTH.,#65365);
#65365=SURFACE_SIDE_STYLE('',(#65370));
#65370=SURFACE_STYLE_FILL_AREA(#65375);
#65375=FILL_AREA_STYLE('Opaque(81,175,227)',(#65380));
#65380=FILL_AREA_STYLE_COLOUR('Opaque(81,175,227)',#65385);
#65385=COLOUR_RGB('Opaque(81,175,227)',0.317647058823529,0.686274509803922,
0.890196078431372);
ENDSEC;
END-ISO-10303-21;
